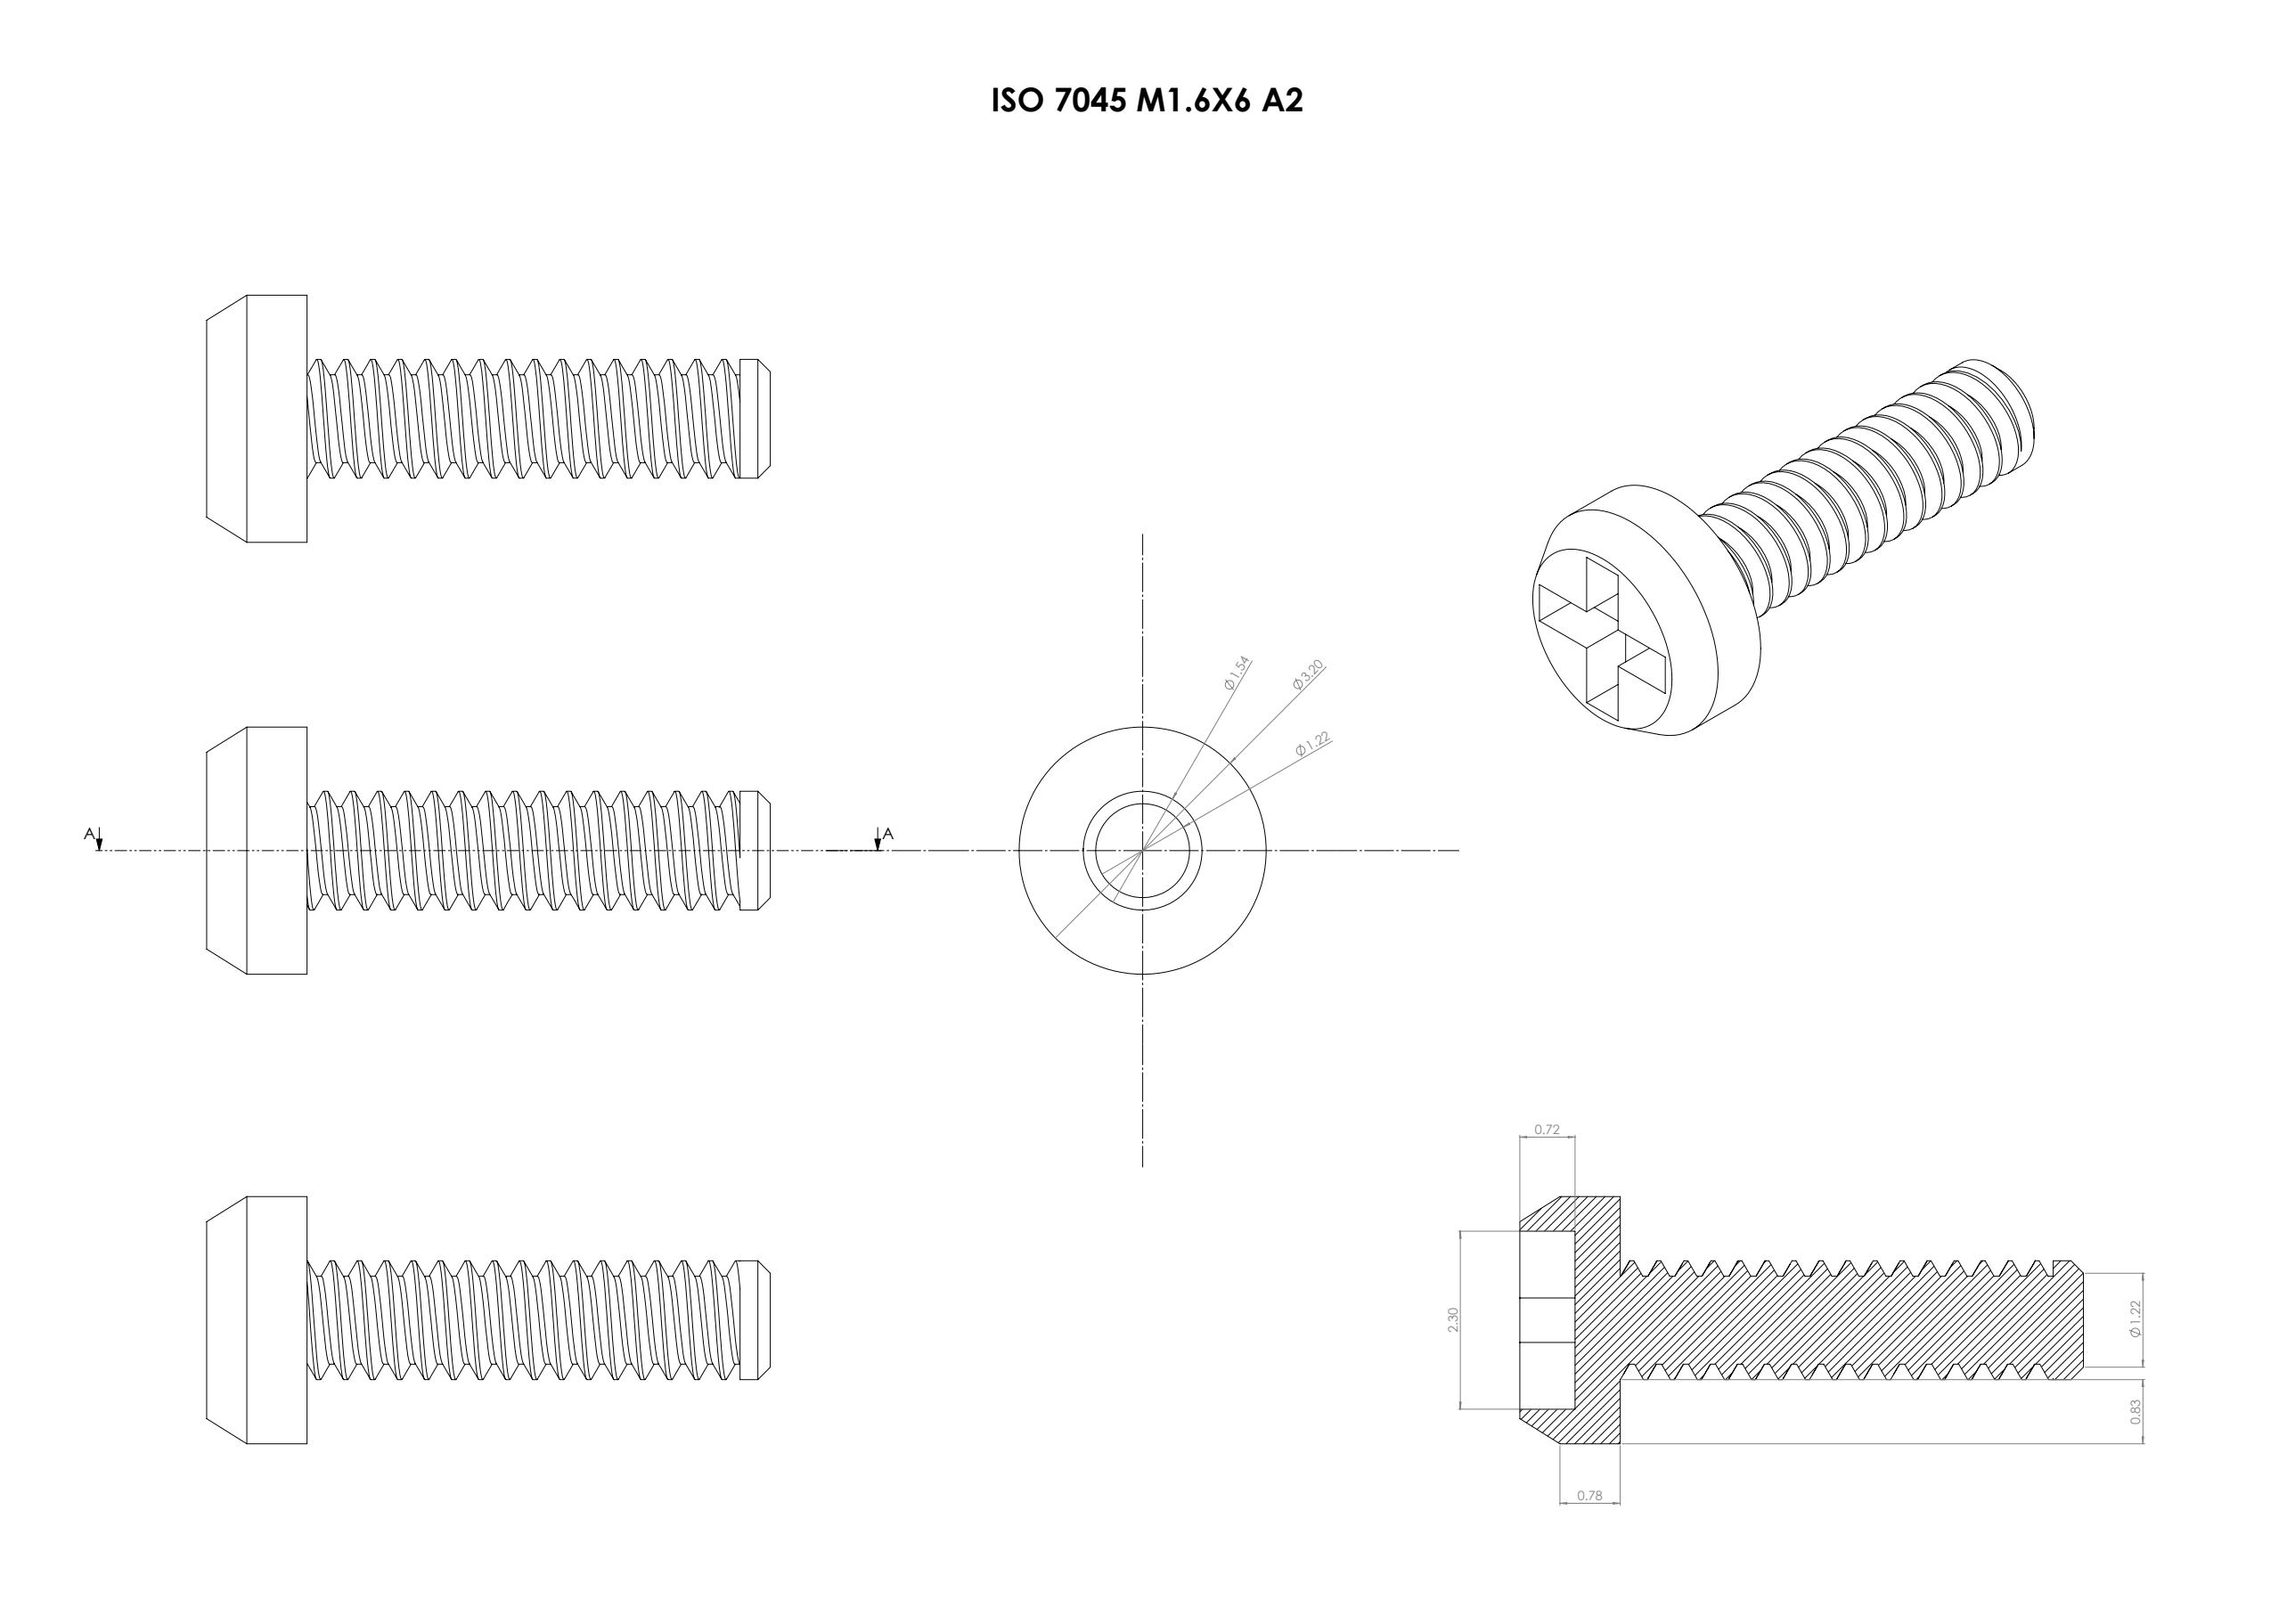
ISO-10303-21;
HEADER;
/* Generated by software containing ST-Developer
 * from STEP Tools, Inc. (www.steptools.com) 
 */

FILE_DESCRIPTION(
/* description */ (''),
/* implementation_level */ '2;1');

FILE_NAME(
/* name */ '19_ISO_7045_M1.6x6_A2.step',
/* time_stamp */ '2026-10-19T23:00:43-07:00',
/* author */ (''),
/* organization */ (''),
/* preprocessor_version */ 'ST-DEVELOPER v20.2',
/* originating_system */ 'Autodesk Translation Framework v15.15.0.0',
/* authorisation */ '');

FILE_SCHEMA (('AUTOMOTIVE_DESIGN { 1 0 10303 214 3 1 1 }'));
ENDSEC;

DATA;
#10=MECHANICAL_DESIGN_GEOMETRIC_PRESENTATION_REPRESENTATION('',(#1015),#55002);
#482=B_SPLINE_SURFACE_WITH_KNOTS('',3,3,((#53741,#53742,#53743,#53744,#53745,
#53746,#53747,#53748,#53749,#53750,#53751,#53752,#53753,#53754,#53755,#53756,
#53757,#53758,#53759,#53760,#53761,#53762,#53763,#53764,#53765,#53766,#53767,
#53768,#53769,#53770,#53771,#53772,#53773,#53774,#53775,#53776,#53777,#53778,
#53779,#53780,#53781,#53782,#53783,#53784,#53785,#53786,#53787,#53788,#53789,
#53790,#53791,#53792,#53793,#53794,#53795,#53796,#53797,#53798,#53799,#53800,
#53801,#53802,#53803,#53804,#53805,#53806,#53807,#53808,#53809,#53810,#53811,
#53812,#53813,#53814,#53815,#53816,#53817,#53818,#53819,#53820,#53821,#53822,
#53823,#53824,#53825,#53826,#53827,#53828,#53829,#53830,#53831,#53832,#53833,
#53834,#53835,#53836,#53837,#53838,#53839,#53840,#53841,#53842,#53843,#53844,
#53845,#53846),(#53847,#53848,#53849,#53850,#53851,#53852,#53853,#53854,
#53855,#53856,#53857,#53858,#53859,#53860,#53861,#53862,#53863,#53864,#53865,
#53866,#53867,#53868,#53869,#53870,#53871,#53872,#53873,#53874,#53875,#53876,
#53877,#53878,#53879,#53880,#53881,#53882,#53883,#53884,#53885,#53886,#53887,
#53888,#53889,#53890,#53891,#53892,#53893,#53894,#53895,#53896,#53897,#53898,
#53899,#53900,#53901,#53902,#53903,#53904,#53905,#53906,#53907,#53908,#53909,
#53910,#53911,#53912,#53913,#53914,#53915,#53916,#53917,#53918,#53919,#53920,
#53921,#53922,#53923,#53924,#53925,#53926,#53927,#53928,#53929,#53930,#53931,
#53932,#53933,#53934,#53935,#53936,#53937,#53938,#53939,#53940,#53941,#53942,
#53943,#53944,#53945,#53946,#53947,#53948,#53949,#53950,#53951,#53952),
(#53953,#53954,#53955,#53956,#53957,#53958,#53959,#53960,#53961,#53962,
#53963,#53964,#53965,#53966,#53967,#53968,#53969,#53970,#53971,#53972,#53973,
#53974,#53975,#53976,#53977,#53978,#53979,#53980,#53981,#53982,#53983,#53984,
#53985,#53986,#53987,#53988,#53989,#53990,#53991,#53992,#53993,#53994,#53995,
#53996,#53997,#53998,#53999,#54000,#54001,#54002,#54003,#54004,#54005,#54006,
#54007,#54008,#54009,#54010,#54011,#54012,#54013,#54014,#54015,#54016,#54017,
#54018,#54019,#54020,#54021,#54022,#54023,#54024,#54025,#54026,#54027,#54028,
#54029,#54030,#54031,#54032,#54033,#54034,#54035,#54036,#54037,#54038,#54039,
#54040,#54041,#54042,#54043,#54044,#54045,#54046,#54047,#54048,#54049,#54050,
#54051,#54052,#54053,#54054,#54055,#54056,#54057,#54058),(#54059,#54060,
#54061,#54062,#54063,#54064,#54065,#54066,#54067,#54068,#54069,#54070,#54071,
#54072,#54073,#54074,#54075,#54076,#54077,#54078,#54079,#54080,#54081,#54082,
#54083,#54084,#54085,#54086,#54087,#54088,#54089,#54090,#54091,#54092,#54093,
#54094,#54095,#54096,#54097,#54098,#54099,#54100,#54101,#54102,#54103,#54104,
#54105,#54106,#54107,#54108,#54109,#54110,#54111,#54112,#54113,#54114,#54115,
#54116,#54117,#54118,#54119,#54120,#54121,#54122,#54123,#54124,#54125,#54126,
#54127,#54128,#54129,#54130,#54131,#54132,#54133,#54134,#54135,#54136,#54137,
#54138,#54139,#54140,#54141,#54142,#54143,#54144,#54145,#54146,#54147,#54148,
#54149,#54150,#54151,#54152,#54153,#54154,#54155,#54156,#54157,#54158,#54159,
#54160,#54161,#54162,#54163,#54164)),.UNSPECIFIED.,.F.,.F.,.F.,(4,4),(4,
1,1,1,1,1,1,1,1,1,1,1,1,1,1,1,1,1,1,1,1,1,1,1,1,1,1,1,1,1,1,1,1,1,1,1,1,
1,1,1,1,1,1,1,1,1,1,1,1,1,1,1,1,1,1,1,1,1,1,1,1,1,1,1,1,1,1,1,1,1,1,1,1,
1,1,1,1,1,1,1,1,1,1,1,1,1,1,1,1,1,1,1,1,1,1,1,1,1,1,1,1,1,1,4),(0.,0.0230940107675851),
(12.4478189520753,13.4453674388536,14.4429159256318,15.4404644124101,16.4380128991884,
17.4355613859667,18.433109872745,19.4306583595232,20.4282068463015,21.4257553330798,
22.423303819858,23.4208523066363,24.4184007934146,25.4159492801929,26.4134977669712,
27.4110462537494,28.4085947405277,29.406143227306,30.4036917140842,31.4012402008625,
32.3987886876408,33.3963371744191,34.3938856611974,35.3914341479756,36.3889826347539,
37.3865311215322,38.3840796083105,39.3816280950887,40.379176581867,41.3767250686453,
42.3742735554236,43.3718220422018,44.3693705289801,45.3669190157584,46.3644675025367,
47.3620159893149,48.3595644760932,49.3571129628715,50.3546614496498,51.352209936428,
52.3497584232063,53.3473069099846,54.3448553967629,55.3424038835411,56.3399523703194,
57.3375008570977,58.335049343876,59.3325978306542,60.3301463174325,61.3276948042108,
62.3252432909891,63.3227917777673,64.3203402645456,65.3178887513239,66.3154372381021,
67.3129857248804,68.3105342116587,69.308082698437,70.3056311852153,71.3031796719935,
72.3007281587718,73.2982766455501,74.2958251323284,75.2933736191066,76.2909221058849,
77.2884705926632,78.2860190794415,79.2835675662197,80.281116052998,81.2786645397763,
82.2762130265546,83.2737615133328,84.2713100001111,85.2688584868894,86.2664069736677,
87.2639554604459,88.2615039472242,89.2590524340025,90.2566009207808,91.254149407559,
92.2516978943373,93.2492463811156,94.2467948678939,95.2443433546721,96.2418918414504,
97.2394403282287,98.236988815007,99.2345373017852,100.232085788564,101.229634275342,
102.22718276212,103.224731248898,104.222279735677,105.219828222455,106.217376709233,
107.214925196011,108.21247368279,109.210022169568,110.207570656346,111.205119143125,
112.202667629903,113.200216116681,114.197764603459,115.195313090238),
 .UNSPECIFIED.);
#483=B_SPLINE_SURFACE_WITH_KNOTS('',3,3,((#54329,#54330,#54331,#54332,#54333,
#54334,#54335,#54336,#54337,#54338,#54339,#54340,#54341,#54342,#54343,#54344,
#54345,#54346,#54347,#54348,#54349,#54350,#54351,#54352,#54353,#54354,#54355,
#54356,#54357,#54358,#54359,#54360,#54361,#54362,#54363,#54364,#54365,#54366,
#54367,#54368,#54369,#54370,#54371,#54372,#54373,#54374,#54375,#54376,#54377,
#54378,#54379,#54380,#54381,#54382,#54383,#54384,#54385,#54386,#54387,#54388,
#54389,#54390,#54391,#54392,#54393,#54394,#54395,#54396,#54397,#54398,#54399,
#54400,#54401,#54402,#54403,#54404,#54405,#54406,#54407,#54408,#54409,#54410,
#54411,#54412,#54413,#54414,#54415,#54416,#54417,#54418,#54419,#54420,#54421,
#54422,#54423,#54424,#54425,#54426,#54427,#54428,#54429,#54430,#54431,#54432,
#54433,#54434),(#54435,#54436,#54437,#54438,#54439,#54440,#54441,#54442,
#54443,#54444,#54445,#54446,#54447,#54448,#54449,#54450,#54451,#54452,#54453,
#54454,#54455,#54456,#54457,#54458,#54459,#54460,#54461,#54462,#54463,#54464,
#54465,#54466,#54467,#54468,#54469,#54470,#54471,#54472,#54473,#54474,#54475,
#54476,#54477,#54478,#54479,#54480,#54481,#54482,#54483,#54484,#54485,#54486,
#54487,#54488,#54489,#54490,#54491,#54492,#54493,#54494,#54495,#54496,#54497,
#54498,#54499,#54500,#54501,#54502,#54503,#54504,#54505,#54506,#54507,#54508,
#54509,#54510,#54511,#54512,#54513,#54514,#54515,#54516,#54517,#54518,#54519,
#54520,#54521,#54522,#54523,#54524,#54525,#54526,#54527,#54528,#54529,#54530,
#54531,#54532,#54533,#54534,#54535,#54536,#54537,#54538,#54539,#54540),
(#54541,#54542,#54543,#54544,#54545,#54546,#54547,#54548,#54549,#54550,
#54551,#54552,#54553,#54554,#54555,#54556,#54557,#54558,#54559,#54560,#54561,
#54562,#54563,#54564,#54565,#54566,#54567,#54568,#54569,#54570,#54571,#54572,
#54573,#54574,#54575,#54576,#54577,#54578,#54579,#54580,#54581,#54582,#54583,
#54584,#54585,#54586,#54587,#54588,#54589,#54590,#54591,#54592,#54593,#54594,
#54595,#54596,#54597,#54598,#54599,#54600,#54601,#54602,#54603,#54604,#54605,
#54606,#54607,#54608,#54609,#54610,#54611,#54612,#54613,#54614,#54615,#54616,
#54617,#54618,#54619,#54620,#54621,#54622,#54623,#54624,#54625,#54626,#54627,
#54628,#54629,#54630,#54631,#54632,#54633,#54634,#54635,#54636,#54637,#54638,
#54639,#54640,#54641,#54642,#54643,#54644,#54645,#54646),(#54647,#54648,
#54649,#54650,#54651,#54652,#54653,#54654,#54655,#54656,#54657,#54658,#54659,
#54660,#54661,#54662,#54663,#54664,#54665,#54666,#54667,#54668,#54669,#54670,
#54671,#54672,#54673,#54674,#54675,#54676,#54677,#54678,#54679,#54680,#54681,
#54682,#54683,#54684,#54685,#54686,#54687,#54688,#54689,#54690,#54691,#54692,
#54693,#54694,#54695,#54696,#54697,#54698,#54699,#54700,#54701,#54702,#54703,
#54704,#54705,#54706,#54707,#54708,#54709,#54710,#54711,#54712,#54713,#54714,
#54715,#54716,#54717,#54718,#54719,#54720,#54721,#54722,#54723,#54724,#54725,
#54726,#54727,#54728,#54729,#54730,#54731,#54732,#54733,#54734,#54735,#54736,
#54737,#54738,#54739,#54740,#54741,#54742,#54743,#54744,#54745,#54746,#54747,
#54748,#54749,#54750,#54751,#54752)),.UNSPECIFIED.,.F.,.F.,.F.,(4,4),(4,
1,1,1,1,1,1,1,1,1,1,1,1,1,1,1,1,1,1,1,1,1,1,1,1,1,1,1,1,1,1,1,1,1,1,1,1,
1,1,1,1,1,1,1,1,1,1,1,1,1,1,1,1,1,1,1,1,1,1,1,1,1,1,1,1,1,1,1,1,1,1,1,1,
1,1,1,1,1,1,1,1,1,1,1,1,1,1,1,1,1,1,1,1,1,1,1,1,1,1,1,1,1,1,4),(0.,0.0230940107675851),
(15.755244690395,16.7527931771733,17.7503416639516,18.7478901507299,19.7454386375081,
20.7429871242864,21.7405356110647,22.738084097843,23.7356325846212,24.7331810713995,
25.7307295581778,26.7282780449561,27.7258265317343,28.7233750185126,29.7209235052909,
30.7184719920692,31.7160204788475,32.7135689656257,33.711117452404,34.7086659391823,
35.7062144259606,36.7037629127388,37.7013113995171,38.6988598862954,39.6964083730737,
40.6939568598519,41.6915053466302,42.6890538334085,43.6866023201868,44.684150806965,
45.6816992937433,46.6792477805216,47.6767962672999,48.6743447540781,49.6718932408564,
50.6694417276347,51.666990214413,52.6645387011912,53.6620871879695,54.6596356747478,
55.6571841615261,56.6547326483043,57.6522811350826,58.6498296218609,59.6473781086392,
60.6449265954174,61.6424750821957,62.640023568974,63.6375720557523,64.6351205425305,
65.6326690293088,66.6302175160871,67.6277660028654,68.6253144896436,69.6228629764219,
70.6204114632002,71.6179599499785,72.6155084367567,73.613056923535,74.6106054103133,
75.6081538970916,76.6057023838698,77.6032508706481,78.6007993574264,79.5983478442047,
80.595896330983,81.5934448177612,82.5909933045395,83.5885417913178,84.5860902780961,
85.5836387648743,86.5811872516526,87.5787357384309,88.5762842252092,89.5738327119874,
90.5713811987657,91.568929685544,92.5664781723222,93.5640266591005,94.5615751458788,
95.5591236326571,96.5566721194354,97.5542206062136,98.5517690929919,99.5493175797702,
100.546866066548,101.544414553327,102.541963040105,103.539511526883,104.537060013662,
105.53460850044,106.532156987218,107.529705473996,108.527253960775,109.524802447553,
110.522350934331,111.519899421109,112.517447907888,113.514996394666,114.512544881444,
115.510093368223,116.507641855001,117.505190341779,118.502738828557),
 .UNSPECIFIED.);
#882=B_SPLINE_CURVE_WITH_KNOTS('',3,(#52556,#52557,#52558,#52559,#52560,
#52561,#52562,#52563,#52564,#52565,#52566,#52567,#52568,#52569,#52570,#52571),
 .UNSPECIFIED.,.F.,.F.,(4,3,3,3,3,4),(-6.23590388473343,-5.98529092066965,
-4.98774243389138,-3.9901939471131,-2.99264546033482,-2.07291355912486),
 .UNSPECIFIED.);
#883=B_SPLINE_CURVE_WITH_KNOTS('',3,(#52579,#52580,#52581,#52582,#52583,
#52584,#52585,#52586,#52587,#52588,#52589,#52590,#52591),.UNSPECIFIED.,
 .F.,.F.,(4,3,3,3,4),(0.,0.997548486778257,1.99509697355654,2.99264546033483,
3.26014431587347),.UNSPECIFIED.);
#884=B_SPLINE_CURVE_WITH_KNOTS('',3,(#52596,#52597,#52598,#52599,#52600,
#52601,#52602,#52603,#52604,#52605,#52606,#52607,#52608,#52609,#52610,#52611,
#52612,#52613,#52614,#52615,#52616,#52617),.UNSPECIFIED.,.F.,.F.,(4,3,3,
3,3,3,3,4),(-12.519089191913,-11.9705818413393,-10.973033354561,-9.97548486778276,
-8.97793638100448,-7.9803878942262,-6.98283940744793,-6.23590388473343),
 .UNSPECIFIED.);
#885=B_SPLINE_CURVE_WITH_KNOTS('',3,(#52618,#52619,#52620,#52621,#52622,
#52623,#52624,#52625,#52626,#52627,#52628,#52629,#52630,#52631,#52632,#52633,
#52634,#52635,#52636,#52637,#52638,#52639),.UNSPECIFIED.,.F.,.F.,(4,3,3,
3,3,3,3,4),(3.26014431587347,3.99019394711311,4.98774243389138,5.98529092066965,
6.98283940744792,7.9803878942262,8.97793638100447,9.54332962305307),
 .UNSPECIFIED.);
#886=B_SPLINE_CURVE_WITH_KNOTS('',3,(#52644,#52645,#52646,#52647,#52648,
#52649,#52650,#52651,#52652,#52653,#52654,#52655,#52656,#52657,#52658,#52659,
#52660,#52661,#52662,#52663,#52664,#52665),.UNSPECIFIED.,.F.,.F.,(4,3,3,
3,3,3,3,4),(-18.8022744990926,-17.955872762009,-16.9583242752307,-15.9607757884524,
-14.9632273016741,-13.9656788148959,-12.9681303281176,-12.519089191913),
 .UNSPECIFIED.);
#887=B_SPLINE_CURVE_WITH_KNOTS('',3,(#52666,#52667,#52668,#52669,#52670,
#52671,#52672,#52673,#52674,#52675,#52676,#52677,#52678,#52679,#52680,#52681,
#52682,#52683,#52684,#52685,#52686,#52687),.UNSPECIFIED.,.F.,.F.,(4,3,3,
3,3,3,3,4),(9.54332962305307,9.97548486778275,10.973033354561,11.9705818413393,
12.9681303281176,13.9656788148959,14.9632273016741,15.8265149302327),
 .UNSPECIFIED.);
#888=B_SPLINE_CURVE_WITH_KNOTS('',3,(#52692,#52693,#52694,#52695,#52696,
#52697,#52698,#52699,#52700,#52701,#52702,#52703,#52704,#52705,#52706,#52707,
#52708,#52709,#52710,#52711,#52712,#52713,#52714,#52715,#52716),
 .UNSPECIFIED.,.F.,.F.,(4,3,3,3,3,3,3,3,4),(-25.0854598062722,-24.9387121694569,
-23.9411636826786,-22.9436151959003,-21.9460667091221,-20.9485182223438,
-19.9509697355655,-18.9534212487872,-18.8022744990926),.UNSPECIFIED.);
#889=B_SPLINE_CURVE_WITH_KNOTS('',3,(#52717,#52718,#52719,#52720,#52721,
#52722,#52723,#52724,#52725,#52726,#52727,#52728,#52729,#52730,#52731,#52732,
#52733,#52734,#52735,#52736,#52737,#52738,#52739,#52740,#52741),
 .UNSPECIFIED.,.F.,.F.,(4,3,3,3,3,3,3,3,4),(15.8265149302327,15.9607757884524,
16.9583242752307,17.955872762009,18.9534212487872,19.9509697355655,20.9485182223438,
21.9460667091221,22.1097002374122),.UNSPECIFIED.);
#890=B_SPLINE_CURVE_WITH_KNOTS('',3,(#52746,#52747,#52748,#52749,#52750,
#52751,#52752,#52753,#52754,#52755,#52756,#52757,#52758,#52759,#52760,#52761,
#52762,#52763,#52764,#52765,#52766,#52767),.UNSPECIFIED.,.F.,.F.,(4,3,3,
3,3,3,3,4),(-31.3686451134518,-30.9240030901265,-29.9264546033483,-28.92890611657,
-27.9313576297917,-26.9338091430134,-25.9362606562352,-25.0854598062722),
 .UNSPECIFIED.);
#891=B_SPLINE_CURVE_WITH_KNOTS('',3,(#52768,#52769,#52770,#52771,#52772,
#52773,#52774,#52775,#52776,#52777,#52778,#52779,#52780,#52781,#52782,#52783,
#52784,#52785,#52786,#52787,#52788,#52789),.UNSPECIFIED.,.F.,.F.,(4,3,3,
3,3,3,3,4),(22.1097002374122,22.9436151959003,23.9411636826786,24.9387121694569,
25.9362606562352,26.9338091430134,27.9313576297917,28.3928855445918),
 .UNSPECIFIED.);
#892=B_SPLINE_CURVE_WITH_KNOTS('',3,(#52794,#52795,#52796,#52797,#52798,
#52799,#52800,#52801,#52802,#52803,#52804,#52805,#52806,#52807,#52808,#52809,
#52810,#52811,#52812,#52813,#52814,#52815),.UNSPECIFIED.,.F.,.F.,(4,3,3,
3,3,3,3,4),(-37.6518304206314,-36.9092940107962,-35.9117455240179,-34.9141970372396,
-33.9166485504614,-32.9191000636831,-31.9215515769048,-31.3686451134518),
 .UNSPECIFIED.);
#893=B_SPLINE_CURVE_WITH_KNOTS('',3,(#52816,#52817,#52818,#52819,#52820,
#52821,#52822,#52823,#52824,#52825,#52826,#52827,#52828,#52829,#52830,#52831,
#52832,#52833,#52834,#52835,#52836,#52837),.UNSPECIFIED.,.F.,.F.,(4,3,3,
3,3,3,3,4),(28.3928855445918,28.92890611657,29.9264546033483,30.9240030901265,
31.9215515769048,32.9191000636831,33.9166485504614,34.6760708517714),
 .UNSPECIFIED.);
#894=B_SPLINE_CURVE_WITH_KNOTS('',3,(#52842,#52843,#52844,#52845,#52846,
#52847,#52848,#52849,#52850,#52851,#52852,#52853,#52854,#52855,#52856,#52857,
#52858,#52859,#52860,#52861,#52862,#52863,#52864,#52865,#52866),
 .UNSPECIFIED.,.F.,.F.,(4,3,3,3,3,3,3,3,4),(-43.9350157278109,-43.8921334182441,
-42.8945849314659,-41.8970364446876,-40.8994879579093,-39.901939471131,
-38.9043909843527,-37.9068424975745,-37.6518304206314),.UNSPECIFIED.);
#895=B_SPLINE_CURVE_WITH_KNOTS('',3,(#52867,#52868,#52869,#52870,#52871,
#52872,#52873,#52874,#52875,#52876,#52877,#52878,#52879,#52880,#52881,#52882,
#52883,#52884,#52885,#52886,#52887,#52888,#52889,#52890,#52891),
 .UNSPECIFIED.,.F.,.F.,(4,3,3,3,3,3,3,3,4),(34.6760708517714,34.9141970372396,
35.9117455240179,36.9092940107962,37.9068424975745,38.9043909843527,39.901939471131,
40.8994879579093,40.959256158951),.UNSPECIFIED.);
#896=B_SPLINE_CURVE_WITH_KNOTS('',3,(#52896,#52897,#52898,#52899,#52900,
#52901,#52902,#52903,#52904,#52905,#52906,#52907,#52908,#52909,#52910,#52911,
#52912,#52913,#52914,#52915,#52916,#52917),.UNSPECIFIED.,.F.,.F.,(4,3,3,
3,3,3,3,4),(-50.2182010349905,-49.8774243389138,-48.8798758521355,-47.8823273653572,
-46.8847788785789,-45.8872303918007,-44.8896819050224,-43.9350157278109),
 .UNSPECIFIED.);
#897=B_SPLINE_CURVE_WITH_KNOTS('',3,(#52918,#52919,#52920,#52921,#52922,
#52923,#52924,#52925,#52926,#52927,#52928,#52929,#52930,#52931,#52932,#52933,
#52934,#52935,#52936,#52937,#52938,#52939),.UNSPECIFIED.,.F.,.F.,(4,3,3,
3,3,3,3,4),(40.959256158951,41.8970364446876,42.8945849314658,43.8921334182441,
44.8896819050224,45.8872303918007,46.8847788785789,47.2424414661306),
 .UNSPECIFIED.);
#898=B_SPLINE_CURVE_WITH_KNOTS('',3,(#52944,#52945,#52946,#52947,#52948,
#52949,#52950,#52951,#52952,#52953,#52954,#52955,#52956,#52957,#52958,#52959,
#52960,#52961,#52962,#52963,#52964,#52965),.UNSPECIFIED.,.F.,.F.,(4,3,3,
3,3,3,3,4),(-56.5013863421701,-55.8627152595834,-54.8651667728052,-53.8676182860269,
-52.8700697992486,-51.8725213124703,-50.874972825692,-50.2182010349905),
 .UNSPECIFIED.);
#899=B_SPLINE_CURVE_WITH_KNOTS('',3,(#52966,#52967,#52968,#52969,#52970,
#52971,#52972,#52973,#52974,#52975,#52976,#52977,#52978,#52979,#52980,#52981,
#52982,#52983,#52984,#52985,#52986,#52987),.UNSPECIFIED.,.F.,.F.,(4,3,3,
3,3,3,3,4),(47.2424414661306,47.8823273653572,48.8798758521355,49.8774243389137,
50.874972825692,51.8725213124703,52.8700697992486,53.5256267733102),
 .UNSPECIFIED.);
#900=B_SPLINE_CURVE_WITH_KNOTS('',3,(#52992,#52993,#52994,#52995,#52996,
#52997,#52998,#52999,#53000,#53001,#53002,#53003,#53004,#53005,#53006,#53007,
#53008,#53009,#53010,#53011,#53012,#53013),.UNSPECIFIED.,.F.,.F.,(4,3,3,
3,3,3,3,4),(-62.7845716493497,-61.8480061802531,-60.8504576934748,-59.8529092066965,
-58.8553607199183,-57.85781223314,-56.8602637463617,-56.5013863421701),
 .UNSPECIFIED.);
#901=B_SPLINE_CURVE_WITH_KNOTS('',3,(#53014,#53015,#53016,#53017,#53018,
#53019,#53020,#53021,#53022,#53023,#53024,#53025,#53026,#53027,#53028,#53029,
#53030,#53031,#53032,#53033,#53034,#53035),.UNSPECIFIED.,.F.,.F.,(4,3,3,
3,3,3,3,4),(53.5256267733102,53.8676182860269,54.8651667728051,55.8627152595834,
56.8602637463617,57.85781223314,58.8553607199182,59.8088120804898),
 .UNSPECIFIED.);
#902=B_SPLINE_CURVE_WITH_KNOTS('',3,(#53040,#53041,#53042,#53043,#53044,
#53045,#53046,#53047,#53048,#53049,#53050,#53051,#53052,#53053,#53054,#53055,
#53056,#53057,#53058,#53059,#53060,#53061,#53062,#53063,#53064),
 .UNSPECIFIED.,.F.,.F.,(4,3,3,3,3,3,3,3,4),(-69.0677569565293,-68.830845587701,
-67.8332971009227,-66.8357486141444,-65.8382001273662,-64.8406516405879,
-63.8431031538096,-62.8455546670314,-62.7845716493497),.UNSPECIFIED.);
#903=B_SPLINE_CURVE_WITH_KNOTS('',3,(#53065,#53066,#53067,#53068,#53069,
#53070,#53071,#53072,#53073,#53074,#53075,#53076,#53077,#53078,#53079,#53080,
#53081,#53082,#53083,#53084,#53085,#53086,#53087,#53088,#53089),
 .UNSPECIFIED.,.F.,.F.,(4,3,3,3,3,3,3,3,4),(59.8088120804898,59.8529092066965,
60.8504576934748,61.8480061802531,62.8455546670313,63.8431031538096,64.8406516405879,
65.8382001273662,66.0919973876694),.UNSPECIFIED.);
#904=B_SPLINE_CURVE_WITH_KNOTS('',3,(#53094,#53095,#53096,#53097,#53098,
#53099,#53100,#53101,#53102,#53103,#53104,#53105,#53106,#53107,#53108,#53109,
#53110,#53111,#53112,#53113,#53114,#53115),.UNSPECIFIED.,.F.,.F.,(4,3,3,
3,3,3,3,4),(-75.3509422637089,-74.8161365083707,-73.8185880215924,-72.8210395348141,
-71.8234910480358,-70.8259425612576,-69.8283940744793,-69.0677569565293),
 .UNSPECIFIED.);
#905=B_SPLINE_CURVE_WITH_KNOTS('',3,(#53116,#53117,#53118,#53119,#53120,
#53121,#53122,#53123,#53124,#53125,#53126,#53127,#53128,#53129,#53130,#53131,
#53132,#53133,#53134,#53135,#53136,#53137),.UNSPECIFIED.,.F.,.F.,(4,3,3,
3,3,3,3,4),(66.0919973876694,66.8357486141444,67.8332971009227,68.830845587701,
69.8283940744792,70.8259425612575,71.8234910480358,72.375182694849),
 .UNSPECIFIED.);
#906=B_SPLINE_CURVE_WITH_KNOTS('',3,(#53142,#53143,#53144,#53145,#53146,
#53147,#53148,#53149,#53150,#53151,#53152,#53153,#53154,#53155,#53156,#53157,
#53158,#53159,#53160,#53161,#53162,#53163),.UNSPECIFIED.,.F.,.F.,(4,3,3,
3,3,3,3,4),(-81.6341275708885,-80.8014274290403,-79.803878942262,-78.8063304554838,
-77.8087819687055,-76.8112334819272,-75.8136849951489,-75.3509422637089),
 .UNSPECIFIED.);
#907=B_SPLINE_CURVE_WITH_KNOTS('',3,(#53164,#53165,#53166,#53167,#53168,
#53169,#53170,#53171,#53172,#53173,#53174,#53175,#53176,#53177,#53178,#53179,
#53180,#53181,#53182,#53183,#53184,#53185),.UNSPECIFIED.,.F.,.F.,(4,3,3,
3,3,3,3,4),(72.375182694849,72.8210395348141,73.8185880215924,74.8161365083706,
75.8136849951489,76.8112334819272,77.8087819687055,78.6583680020286),
 .UNSPECIFIED.);
#908=B_SPLINE_CURVE_WITH_KNOTS('',3,(#53190,#53191,#53192,#53193,#53194,
#53195,#53196,#53197,#53198,#53199,#53200,#53201,#53202,#53203,#53204,#53205,
#53206,#53207,#53208,#53209,#53210,#53211,#53212,#53213,#53214),
 .UNSPECIFIED.,.F.,.F.,(4,3,3,3,3,3,3,3,4),(-87.9173128780681,-87.7842668364882,
-86.78671834971,-85.7891698629317,-84.7916213761534,-83.7940728893752,-82.7965244025969,
-81.7989759158186,-81.6341275708885),.UNSPECIFIED.);
#909=B_SPLINE_CURVE_WITH_KNOTS('',3,(#53215,#53216,#53217,#53218,#53219,
#53220,#53221,#53222,#53223,#53224,#53225,#53226,#53227,#53228,#53229,#53230,
#53231,#53232,#53233,#53234,#53235,#53236,#53237,#53238,#53239),
 .UNSPECIFIED.,.F.,.F.,(4,3,3,3,3,3,3,3,4),(78.6583680020286,78.8063304554837,
79.803878942262,80.8014274290403,81.7989759158185,82.7965244025968,83.7940728893751,
84.7916213761534,84.9415533092082),.UNSPECIFIED.);
#910=B_SPLINE_CURVE_WITH_KNOTS('',3,(#53244,#53245,#53246,#53247,#53248,
#53249,#53250,#53251,#53252,#53253,#53254,#53255,#53256,#53257,#53258,#53259,
#53260,#53261,#53262,#53263,#53264,#53265),.UNSPECIFIED.,.F.,.F.,(4,3,3,
3,3,3,3,4),(-94.2004981852477,-93.7695577571579,-92.7720092703796,-91.7744607836013,
-90.7769122968231,-89.7793638100448,-88.7818153232665,-87.9173128780681),
 .UNSPECIFIED.);
#911=B_SPLINE_CURVE_WITH_KNOTS('',3,(#53266,#53267,#53268,#53269,#53270,
#53271,#53272,#53273,#53274,#53275,#53276,#53277,#53278,#53279,#53280,#53281,
#53282,#53283,#53284,#53285,#53286,#53287),.UNSPECIFIED.,.F.,.F.,(4,3,3,
3,3,3,3,4),(84.9415533092082,85.7891698629316,86.7867183497099,87.7842668364882,
88.7818153232665,89.7793638100448,90.776912296823,91.2247386163878),
 .UNSPECIFIED.);
#912=B_SPLINE_CURVE_WITH_KNOTS('',3,(#53292,#53293,#53294,#53295,#53296,
#53297,#53298,#53299,#53300,#53301,#53302,#53303,#53304,#53305,#53306,#53307,
#53308,#53309,#53310,#53311,#53312,#53313),.UNSPECIFIED.,.F.,.F.,(4,3,3,
3,3,3,3,4),(-100.483683492427,-99.7548486778276,-98.7573001910493,-97.759751704271,
-96.7622032174927,-95.7646547307145,-94.7671062439362,-94.2004981852477),
 .UNSPECIFIED.);
#913=B_SPLINE_CURVE_WITH_KNOTS('',3,(#53314,#53315,#53316,#53317,#53318,
#53319,#53320,#53321,#53322,#53323,#53324,#53325,#53326,#53327,#53328,#53329,
#53330,#53331,#53332,#53333,#53334,#53335),.UNSPECIFIED.,.F.,.F.,(4,3,3,
3,3,3,3,4),(91.2247386163878,91.7744607836013,92.7720092703796,93.7695577571579,
94.7671062439361,95.7646547307144,96.7622032174927,97.5079239235673),
 .UNSPECIFIED.);
#914=B_SPLINE_CURVE_WITH_KNOTS('',3,(#53341,#53342,#53343,#53344),
 .UNSPECIFIED.,.F.,.F.,(4,4),(116.238928182822,116.429825269433),
 .UNSPECIFIED.);
#915=B_SPLINE_CURVE_WITH_KNOTS('',3,(#53350,#53351,#53352,#53353,#53354,
#53355,#53356,#53357,#53358,#53359),.UNSPECIFIED.,.F.,.F.,(4,1,1,1,1,1,
1,4),(109.955742875643,110.522350934331,111.519899421109,112.517447907888,
113.514996394666,114.512544881444,115.510093368223,116.238928182822),
 .UNSPECIFIED.);
#916=B_SPLINE_CURVE_WITH_KNOTS('',3,(#53362,#53363,#53364,#53365,#53366,
#53367,#53368,#53369,#53370),.UNSPECIFIED.,.F.,.F.,(4,1,1,1,1,1,4),(109.955742875643,
110.207570656346,111.205119143125,112.202667629903,113.200216116681,114.197764603459,
115.195313090238),.UNSPECIFIED.);
#917=B_SPLINE_CURVE_WITH_KNOTS('',3,(#53375,#53376,#53377,#53378,#53379,
#53380,#53381,#53382,#53383,#53384),.UNSPECIFIED.,.F.,.F.,(4,1,1,1,1,1,
1,4),(103.672557568463,104.537060013662,105.53460850044,106.532156987218,
107.529705473996,108.527253960775,109.524802447553,109.955742875643),
 .UNSPECIFIED.);
#918=B_SPLINE_CURVE_WITH_KNOTS('',3,(#53385,#53386,#53387,#53388,#53389,
#53390,#53391,#53392,#53393,#53394),.UNSPECIFIED.,.F.,.F.,(4,1,1,1,1,1,
1,4),(103.672557568463,104.222279735677,105.219828222455,106.217376709233,
107.214925196011,108.21247368279,109.210022169568,109.955742875643),
 .UNSPECIFIED.);
#919=B_SPLINE_CURVE_WITH_KNOTS('',3,(#53399,#53400,#53401,#53402,#53403,
#53404,#53405,#53406,#53407,#53408,#53409),.UNSPECIFIED.,.F.,.F.,(4,1,1,
1,1,1,1,1,4),(97.3893722612836,97.5542206062136,98.5517690929919,99.5493175797702,
100.546866066548,101.544414553327,102.541963040105,103.539511526883,103.672557568463),
 .UNSPECIFIED.);
#920=B_SPLINE_CURVE_WITH_KNOTS('',3,(#53410,#53411,#53412,#53413,#53414,
#53415,#53416,#53417,#53418,#53419),.UNSPECIFIED.,.F.,.F.,(4,1,1,1,1,1,
1,4),(97.3893722612836,98.236988815007,99.2345373017852,100.232085788564,
101.229634275342,102.22718276212,103.224731248898,103.672557568463),
 .UNSPECIFIED.);
#921=B_SPLINE_CURVE_WITH_KNOTS('',3,(#53424,#53425,#53426,#53427,#53428,
#53429,#53430,#53431,#53432,#53433),.UNSPECIFIED.,.F.,.F.,(4,1,1,1,1,1,
1,4),(91.106186954104,91.568929685544,92.5664781723222,93.5640266591005,
94.5615751458788,95.5591236326571,96.5566721194354,97.3893722612836),
 .UNSPECIFIED.);
#922=B_SPLINE_CURVE_WITH_KNOTS('',3,(#53434,#53435,#53436,#53437,#53438,
#53439,#53440,#53441,#53442,#53443,#53444),.UNSPECIFIED.,.F.,.F.,(4,1,1,
1,1,1,1,1,4),(91.106186954104,91.254149407559,92.2516978943373,93.2492463811156,
94.2467948678939,95.2443433546721,96.2418918414504,97.2394403282287,97.3893722612836),
 .UNSPECIFIED.);
#923=B_SPLINE_CURVE_WITH_KNOTS('',3,(#53449,#53450,#53451,#53452,#53453,
#53454,#53455,#53456,#53457,#53458),.UNSPECIFIED.,.F.,.F.,(4,1,1,1,1,1,
1,4),(84.8230016469244,85.5836387648743,86.5811872516526,87.5787357384309,
88.5762842252092,89.5738327119874,90.5713811987657,91.106186954104),
 .UNSPECIFIED.);
#924=B_SPLINE_CURVE_WITH_KNOTS('',3,(#53459,#53460,#53461,#53462,#53463,
#53464,#53465,#53466,#53467,#53468),.UNSPECIFIED.,.F.,.F.,(4,1,1,1,1,1,
1,4),(84.8230016469244,85.2688584868894,86.2664069736677,87.2639554604459,
88.2615039472242,89.2590524340025,90.2566009207808,91.106186954104),
 .UNSPECIFIED.);
#925=B_SPLINE_CURVE_WITH_KNOTS('',3,(#53473,#53474,#53475,#53476,#53477,
#53478,#53479,#53480,#53481,#53482,#53483),.UNSPECIFIED.,.F.,.F.,(4,1,1,
1,1,1,1,1,4),(78.5398163397448,78.6007993574264,79.5983478442047,80.595896330983,
81.5934448177612,82.5909933045395,83.5885417913178,84.5860902780961,84.8230016469244),
 .UNSPECIFIED.);
#926=B_SPLINE_CURVE_WITH_KNOTS('',3,(#53484,#53485,#53486,#53487,#53488,
#53489,#53490,#53491,#53492,#53493),.UNSPECIFIED.,.F.,.F.,(4,1,1,1,1,1,
1,4),(78.5398163397448,79.2835675662197,80.281116052998,81.2786645397763,
82.2762130265546,83.2737615133328,84.2713100001111,84.8230016469244),
 .UNSPECIFIED.);
#927=B_SPLINE_CURVE_WITH_KNOTS('',3,(#53498,#53499,#53500,#53501,#53502,
#53503,#53504,#53505,#53506,#53507),.UNSPECIFIED.,.F.,.F.,(4,1,1,1,1,1,
1,4),(72.2566310325652,72.6155084367567,73.613056923535,74.6106054103133,
75.6081538970916,76.6057023838698,77.6032508706481,78.5398163397448),
 .UNSPECIFIED.);
#928=B_SPLINE_CURVE_WITH_KNOTS('',3,(#53508,#53509,#53510,#53511,#53512,
#53513,#53514,#53515,#53516,#53517,#53518),.UNSPECIFIED.,.F.,.F.,(4,1,1,
1,1,1,1,1,4),(72.2566310325652,72.3007281587718,73.2982766455501,74.2958251323284,
75.2933736191066,76.2909221058849,77.2884705926632,78.2860190794415,78.5398163397448),
 .UNSPECIFIED.);
#929=B_SPLINE_CURVE_WITH_KNOTS('',3,(#53523,#53524,#53525,#53526,#53527,
#53528,#53529,#53530,#53531,#53532),.UNSPECIFIED.,.F.,.F.,(4,1,1,1,1,1,
1,4),(65.9734457253856,66.6302175160871,67.6277660028654,68.6253144896436,
69.6228629764219,70.6204114632002,71.6179599499785,72.2566310325652),
 .UNSPECIFIED.);
#930=B_SPLINE_CURVE_WITH_KNOTS('',3,(#53533,#53534,#53535,#53536,#53537,
#53538,#53539,#53540,#53541,#53542),.UNSPECIFIED.,.F.,.F.,(4,1,1,1,1,1,
1,4),(65.9734457253856,66.3154372381021,67.3129857248804,68.3105342116587,
69.308082698437,70.3056311852153,71.3031796719935,72.2566310325652),
 .UNSPECIFIED.);
#931=B_SPLINE_CURVE_WITH_KNOTS('',3,(#53547,#53548,#53549,#53550,#53551,
#53552,#53553,#53554,#53555,#53556),.UNSPECIFIED.,.F.,.F.,(4,1,1,1,1,1,
1,4),(59.690260418206,60.6449265954174,61.6424750821957,62.640023568974,
63.6375720557523,64.6351205425305,65.6326690293088,65.9734457253856),
 .UNSPECIFIED.);
#932=B_SPLINE_CURVE_WITH_KNOTS('',3,(#53557,#53558,#53559,#53560,#53561,
#53562,#53563,#53564,#53565,#53566),.UNSPECIFIED.,.F.,.F.,(4,1,1,1,1,1,
1,4),(59.690260418206,60.3301463174325,61.3276948042108,62.3252432909891,
63.3227917777673,64.3203402645456,65.3178887513239,65.9734457253856),
 .UNSPECIFIED.);
#933=B_SPLINE_CURVE_WITH_KNOTS('',3,(#53571,#53572,#53573,#53574,#53575,
#53576,#53577,#53578,#53579,#53580,#53581),.UNSPECIFIED.,.F.,.F.,(4,1,1,
1,1,1,1,1,4),(53.4070751110265,53.6620871879695,54.6596356747478,55.6571841615261,
56.6547326483043,57.6522811350826,58.6498296218609,59.6473781086392,59.690260418206),
 .UNSPECIFIED.);
#934=B_SPLINE_CURVE_WITH_KNOTS('',3,(#53582,#53583,#53584,#53585,#53586,
#53587,#53588,#53589,#53590,#53591),.UNSPECIFIED.,.F.,.F.,(4,1,1,1,1,1,
1,4),(53.4070751110264,54.3448553967629,55.3424038835411,56.3399523703194,
57.3375008570977,58.335049343876,59.3325978306542,59.690260418206),
 .UNSPECIFIED.);
#935=B_SPLINE_CURVE_WITH_KNOTS('',3,(#53596,#53597,#53598,#53599,#53600,
#53601,#53602,#53603,#53604,#53605),.UNSPECIFIED.,.F.,.F.,(4,1,1,1,1,1,
1,4),(47.1238898038469,47.6767962672999,48.6743447540781,49.6718932408564,
50.6694417276347,51.666990214413,52.6645387011912,53.4070751110265),
 .UNSPECIFIED.);
#936=B_SPLINE_CURVE_WITH_KNOTS('',3,(#53606,#53607,#53608,#53609,#53610,
#53611,#53612,#53613,#53614,#53615,#53616),.UNSPECIFIED.,.F.,.F.,(4,1,1,
1,1,1,1,1,4),(47.1238898038468,47.3620159893149,48.3595644760932,49.3571129628715,
50.3546614496498,51.352209936428,52.3497584232063,53.3473069099846,53.4070751110264),
 .UNSPECIFIED.);
#937=B_SPLINE_CURVE_WITH_KNOTS('',3,(#53621,#53622,#53623,#53624,#53625,
#53626,#53627,#53628,#53629,#53630),.UNSPECIFIED.,.F.,.F.,(4,1,1,1,1,1,
1,4),(40.8407044966673,41.6915053466302,42.6890538334085,43.6866023201868,
44.684150806965,45.6816992937433,46.6792477805216,47.1238898038469),
 .UNSPECIFIED.);
#938=B_SPLINE_CURVE_WITH_KNOTS('',3,(#53631,#53632,#53633,#53634,#53635,
#53636,#53637,#53638,#53639,#53640),.UNSPECIFIED.,.F.,.F.,(4,1,1,1,1,1,
1,4),(40.8407044966672,41.3767250686453,42.3742735554236,43.3718220422018,
44.3693705289801,45.3669190157584,46.3644675025367,47.1238898038468),
 .UNSPECIFIED.);
#939=B_SPLINE_CURVE_WITH_KNOTS('',3,(#53645,#53646,#53647,#53648,#53649,
#53650,#53651,#53652,#53653,#53654,#53655),.UNSPECIFIED.,.F.,.F.,(4,1,1,
1,1,1,1,1,4),(34.5575191894877,34.7086659391823,35.7062144259606,36.7037629127388,
37.7013113995171,38.6988598862954,39.6964083730737,40.6939568598519,40.8407044966673),
 .UNSPECIFIED.);
#940=B_SPLINE_CURVE_WITH_KNOTS('',3,(#53656,#53657,#53658,#53659,#53660,
#53661,#53662,#53663,#53664,#53665),.UNSPECIFIED.,.F.,.F.,(4,1,1,1,1,1,
1,4),(34.5575191894876,35.3914341479756,36.3889826347539,37.3865311215322,
38.3840796083105,39.3816280950887,40.379176581867,40.8407044966672),
 .UNSPECIFIED.);
#941=B_SPLINE_CURVE_WITH_KNOTS('',3,(#53670,#53671,#53672,#53673,#53674,
#53675,#53676,#53677,#53678,#53679),.UNSPECIFIED.,.F.,.F.,(4,1,1,1,1,1,
1,4),(28.2743338823081,28.7233750185126,29.7209235052909,30.7184719920692,
31.7160204788475,32.7135689656257,33.711117452404,34.5575191894877),
 .UNSPECIFIED.);
#942=B_SPLINE_CURVE_WITH_KNOTS('',3,(#53680,#53681,#53682,#53683,#53684,
#53685,#53686,#53687,#53688,#53689,#53690),.UNSPECIFIED.,.F.,.F.,(4,1,1,
1,1,1,1,1,4),(28.274333882308,28.4085947405277,29.406143227306,30.4036917140842,
31.4012402008625,32.3987886876408,33.3963371744191,34.3938856611974,34.5575191894876),
 .UNSPECIFIED.);
#943=B_SPLINE_CURVE_WITH_KNOTS('',3,(#53695,#53696,#53697,#53698,#53699,
#53700,#53701,#53702,#53703,#53704),.UNSPECIFIED.,.F.,.F.,(4,1,1,1,1,1,
1,4),(21.9911485751285,22.738084097843,23.7356325846212,24.7331810713995,
25.7307295581778,26.7282780449561,27.7258265317343,28.2743338823081),
 .UNSPECIFIED.);
#944=B_SPLINE_CURVE_WITH_KNOTS('',3,(#53705,#53706,#53707,#53708,#53709,
#53710,#53711,#53712,#53713,#53714),.UNSPECIFIED.,.F.,.F.,(4,1,1,1,1,1,
1,4),(21.9911485751285,22.423303819858,23.4208523066363,24.4184007934146,
25.4159492801929,26.4134977669712,27.4110462537494,28.274333882308),
 .UNSPECIFIED.);
#945=B_SPLINE_CURVE_WITH_KNOTS('',3,(#53721,#53722,#53723,#53724,#53725,
#53726,#53727,#53728,#53729,#53730),.UNSPECIFIED.,.F.,.F.,(4,1,1,1,1,1,
1,4),(15.755244690395,16.7527931771733,17.7503416639516,18.7478901507299,
19.7454386375081,20.7429871242864,21.7405356110647,21.9911485751285),
 .UNSPECIFIED.);
#946=B_SPLINE_CURVE_WITH_KNOTS('',3,(#53731,#53732,#53733,#53734,#53735,
#53736,#53737,#53738,#53739,#53740),.UNSPECIFIED.,.F.,.F.,(4,1,1,1,1,1,
1,4),(15.7079632679489,16.4380128991884,17.4355613859667,18.433109872745,
19.4306583595232,20.4282068463015,21.4257553330798,21.9911485751285),
 .UNSPECIFIED.);
#947=B_SPLINE_CURVE_WITH_KNOTS('',3,(#54166,#54167,#54168,#54169,#54170,
#54171,#54172,#54173,#54174,#54175,#54176,#54177,#54178,#54179,#54180,#54181,
#54182,#54183,#54184,#54185,#54186,#54187,#54188,#54189,#54190,#54191,#54192,
#54193,#54194,#54195,#54196,#54197,#54198,#54199,#54200,#54201,#54202,#54203,
#54204,#54205,#54206,#54207,#54208,#54209,#54210,#54211),.UNSPECIFIED.,
 .F.,.F.,(4,3,3,3,3,3,3,3,3,3,3,3,3,3,3,4),(-0.140062757837262,-0.134086502655375,
-0.12147120271553,-0.113407421882847,-0.103769248913591,-0.0940394054438087,
-0.077137461601402,-0.0675091408822671,-0.0624229504780978,-0.0526720700183036,
-0.045988001471802,-0.0296865557803863,-0.0231241453191696,-0.0164915301952035,
-0.00152741804160966,0.),.UNSPECIFIED.);
#948=B_SPLINE_CURVE_WITH_KNOTS('',3,(#54212,#54213,#54214,#54215,#54216,
#54217,#54218,#54219,#54220,#54221,#54222,#54223,#54224),.UNSPECIFIED.,
 .F.,.F.,(4,3,3,3,4),(97.5079239235673,97.759751704271,98.7573001910492,
99.7548486778275,100.674580579037),.UNSPECIFIED.);
#949=B_SPLINE_CURVE_WITH_KNOTS('',3,(#54226,#54227,#54228,#54229,#54230,
#54231,#54232,#54233,#54234,#54235,#54236,#54237,#54238,#54239,#54240,#54241,
#54242,#54243,#54244,#54245,#54246,#54247,#54248,#54249,#54250,#54251,#54252,
#54253,#54254,#54255,#54256,#54257,#54258,#54259,#54260,#54261,#54262,#54263,
#54264,#54265,#54266,#54267,#54268,#54269,#54270,#54271,#54272,#54273,#54274),
 .UNSPECIFIED.,.F.,.F.,(4,3,3,3,3,3,3,3,3,3,3,3,3,3,3,3,4),(-0.140969988491055,
-0.136418201281803,-0.126519129074011,-0.119862943924149,-0.108023198611015,
-0.101287865761346,-0.090139871551597,-0.0833947080504807,-0.0768589146704996,
-0.0729154820906274,-0.0587558950229259,-0.0520363404538416,-0.0380581629180643,
-0.0301338231072477,-0.0233108653882379,-0.00436182509706893,0.),
 .UNSPECIFIED.);
#950=B_SPLINE_CURVE_WITH_KNOTS('',3,(#54275,#54276,#54277,#54278,#54279),
 .UNSPECIFIED.,.F.,.F.,(4,1,4),(14.5207325112001,15.4404644124101,15.7079632679489),
 .UNSPECIFIED.);
#951=B_SPLINE_CURVE_WITH_KNOTS('',3,(#54281,#54282,#54283,#54284,#54285,
#54286,#54287,#54288,#54289,#54290,#54291,#54292,#54293,#54294,#54295,#54296,
#54297,#54298,#54299,#54300,#54301,#54302,#54303,#54304,#54305,#54306,#54307,
#54308,#54309,#54310,#54311,#54312,#54313,#54314,#54315,#54316,#54317,#54318,
#54319,#54320,#54321,#54322,#54323,#54324,#54325,#54326),.UNSPECIFIED.,
 .F.,.F.,(4,3,3,3,3,3,3,3,3,3,3,3,3,3,3,4),(-0.140062757837253,-0.134086502655363,
-0.121471201692539,-0.113407420189978,-0.103769238848968,-0.0940394045173825,
-0.077137458468192,-0.0675091411229651,-0.0624229504780945,-0.0526720783361747,
-0.0459880025256372,-0.0296865588875043,-0.0231241679347418,-0.0164915350738677,
-0.00152742707365775,0.),.UNSPECIFIED.);
#952=B_SPLINE_CURVE_WITH_KNOTS('',3,(#54754,#54755,#54756,#54757,#54758,
#54759,#54760,#54761,#54762,#54763,#54764,#54765,#54766,#54767,#54768,#54769,
#54770,#54771,#54772,#54773,#54774,#54775,#54776,#54777,#54778,#54779,#54780,
#54781,#54782,#54783,#54784,#54785,#54786,#54787,#54788,#54789,#54790,#54791,
#54792,#54793,#54794,#54795,#54796,#54797,#54798,#54799,#54800,#54801,#54802),
 .UNSPECIFIED.,.F.,.F.,(4,3,3,3,3,3,3,3,3,3,3,3,3,3,3,3,4),(-0.140969988491055,
-0.136418201281804,-0.12651913264835,-0.119862947097551,-0.108023216524302,
-0.101287867723297,-0.0901398753013339,-0.0833947302596222,-0.0768589166211874,
-0.0729154820906318,-0.0587558981038184,-0.0520363434544736,-0.0380581662283503,
-0.0301338238248305,-0.0233108669968244,-0.00436182790272715,0.),
 .UNSPECIFIED.);
#953=B_SPLINE_CURVE_WITH_KNOTS('',3,(#54803,#54804,#54805,#54806,#54807,
#54808,#54809,#54810,#54811,#54812),.UNSPECIFIED.,.F.,.F.,(4,3,3,4),(-102.747494138162,
-101.749945651384,-100.752397164606,-100.483683492427),.UNSPECIFIED.);
#975=SHAPE_REPRESENTATION_RELATIONSHIP('SRR','None',#55123,#995);
#995=ADVANCED_BREP_SHAPE_REPRESENTATION('',(#1035),#55001);
#1015=STYLED_ITEM('',(#55400),#1035);
#1035=MANIFOLD_SOLID_BREP('ISO_7045_M1.6x6_A2',#24548);
#1274=FACE_BOUND('',#5366,.T.);
#1275=FACE_BOUND('',#5377,.T.);
#1935=PLANE('',#27114);
#1936=PLANE('',#27119);
#1937=PLANE('',#27120);
#1938=PLANE('',#27121);
#1939=PLANE('',#27122);
#1940=PLANE('',#27123);
#1941=PLANE('',#27124);
#1942=PLANE('',#27125);
#1943=PLANE('',#27127);
#1944=PLANE('',#27128);
#1945=PLANE('',#27129);
#1946=PLANE('',#27130);
#1947=PLANE('',#27131);
#1948=PLANE('',#27132);
#1949=PLANE('',#27133);
#1950=PLANE('',#27134);
#1951=PLANE('',#27137);
#2376=CYLINDRICAL_SURFACE('',#27075,0.076925);
#2377=CYLINDRICAL_SURFACE('',#27079,0.076925);
#2378=CYLINDRICAL_SURFACE('',#27080,0.076925);
#2379=CYLINDRICAL_SURFACE('',#27081,0.076925);
#2380=CYLINDRICAL_SURFACE('',#27082,0.076925);
#2381=CYLINDRICAL_SURFACE('',#27083,0.076925);
#2382=CYLINDRICAL_SURFACE('',#27084,0.076925);
#2383=CYLINDRICAL_SURFACE('',#27085,0.076925);
#2384=CYLINDRICAL_SURFACE('',#27086,0.076925);
#2385=CYLINDRICAL_SURFACE('',#27087,0.076925);
#2386=CYLINDRICAL_SURFACE('',#27088,0.076925);
#2387=CYLINDRICAL_SURFACE('',#27089,0.076925);
#2388=CYLINDRICAL_SURFACE('',#27090,0.076925);
#2389=CYLINDRICAL_SURFACE('',#27091,0.076925);
#2390=CYLINDRICAL_SURFACE('',#27092,0.076925);
#2391=CYLINDRICAL_SURFACE('',#27093,0.076925);
#2392=CYLINDRICAL_SURFACE('',#27094,0.056925);
#2393=CYLINDRICAL_SURFACE('',#27096,0.056925);
#2394=CYLINDRICAL_SURFACE('',#27098,0.056925);
#2395=CYLINDRICAL_SURFACE('',#27099,0.056925);
#2396=CYLINDRICAL_SURFACE('',#27100,0.056925);
#2397=CYLINDRICAL_SURFACE('',#27101,0.056925);
#2398=CYLINDRICAL_SURFACE('',#27102,0.056925);
#2399=CYLINDRICAL_SURFACE('',#27103,0.056925);
#2400=CYLINDRICAL_SURFACE('',#27104,0.056925);
#2401=CYLINDRICAL_SURFACE('',#27105,0.056925);
#2402=CYLINDRICAL_SURFACE('',#27106,0.056925);
#2403=CYLINDRICAL_SURFACE('',#27107,0.056925);
#2404=CYLINDRICAL_SURFACE('',#27108,0.056925);
#2405=CYLINDRICAL_SURFACE('',#27109,0.056925);
#2406=CYLINDRICAL_SURFACE('',#27110,0.056925);
#2407=CYLINDRICAL_SURFACE('',#27111,0.056925);
#2408=CYLINDRICAL_SURFACE('',#27112,0.056925);
#2409=CYLINDRICAL_SURFACE('',#27116,0.056925);
#2410=CYLINDRICAL_SURFACE('',#27117,0.076925);
#2411=CYLINDRICAL_SURFACE('',#27139,0.16);
#3719=FACE_OUTER_BOUND('',#5321,.T.);
#3720=FACE_OUTER_BOUND('',#5322,.T.);
#3721=FACE_OUTER_BOUND('',#5323,.T.);
#3722=FACE_OUTER_BOUND('',#5324,.T.);
#3723=FACE_OUTER_BOUND('',#5325,.T.);
#3724=FACE_OUTER_BOUND('',#5326,.T.);
#3725=FACE_OUTER_BOUND('',#5327,.T.);
#3726=FACE_OUTER_BOUND('',#5328,.T.);
#3727=FACE_OUTER_BOUND('',#5329,.T.);
#3728=FACE_OUTER_BOUND('',#5330,.T.);
#3729=FACE_OUTER_BOUND('',#5331,.T.);
#3730=FACE_OUTER_BOUND('',#5332,.T.);
#3731=FACE_OUTER_BOUND('',#5333,.T.);
#3732=FACE_OUTER_BOUND('',#5334,.T.);
#3733=FACE_OUTER_BOUND('',#5335,.T.);
#3734=FACE_OUTER_BOUND('',#5336,.T.);
#3735=FACE_OUTER_BOUND('',#5337,.T.);
#3736=FACE_OUTER_BOUND('',#5338,.T.);
#3737=FACE_OUTER_BOUND('',#5339,.T.);
#3738=FACE_OUTER_BOUND('',#5340,.T.);
#3739=FACE_OUTER_BOUND('',#5341,.T.);
#3740=FACE_OUTER_BOUND('',#5342,.T.);
#3741=FACE_OUTER_BOUND('',#5343,.T.);
#3742=FACE_OUTER_BOUND('',#5344,.T.);
#3743=FACE_OUTER_BOUND('',#5345,.T.);
#3744=FACE_OUTER_BOUND('',#5346,.T.);
#3745=FACE_OUTER_BOUND('',#5347,.T.);
#3746=FACE_OUTER_BOUND('',#5348,.T.);
#3747=FACE_OUTER_BOUND('',#5349,.T.);
#3748=FACE_OUTER_BOUND('',#5350,.T.);
#3749=FACE_OUTER_BOUND('',#5351,.T.);
#3750=FACE_OUTER_BOUND('',#5352,.T.);
#3751=FACE_OUTER_BOUND('',#5353,.T.);
#3752=FACE_OUTER_BOUND('',#5354,.T.);
#3753=FACE_OUTER_BOUND('',#5355,.T.);
#3754=FACE_OUTER_BOUND('',#5356,.T.);
#3755=FACE_OUTER_BOUND('',#5357,.T.);
#3756=FACE_OUTER_BOUND('',#5358,.T.);
#3757=FACE_OUTER_BOUND('',#5359,.T.);
#3758=FACE_OUTER_BOUND('',#5360,.T.);
#3759=FACE_OUTER_BOUND('',#5361,.T.);
#3760=FACE_OUTER_BOUND('',#5362,.T.);
#3761=FACE_OUTER_BOUND('',#5363,.T.);
#3762=FACE_OUTER_BOUND('',#5364,.T.);
#3763=FACE_OUTER_BOUND('',#5365,.T.);
#3764=FACE_OUTER_BOUND('',#5367,.T.);
#3765=FACE_OUTER_BOUND('',#5368,.T.);
#3766=FACE_OUTER_BOUND('',#5369,.T.);
#3767=FACE_OUTER_BOUND('',#5370,.T.);
#3768=FACE_OUTER_BOUND('',#5371,.T.);
#3769=FACE_OUTER_BOUND('',#5372,.T.);
#3770=FACE_OUTER_BOUND('',#5373,.T.);
#3771=FACE_OUTER_BOUND('',#5374,.T.);
#3772=FACE_OUTER_BOUND('',#5375,.T.);
#3773=FACE_OUTER_BOUND('',#5376,.T.);
#3774=FACE_OUTER_BOUND('',#5378,.T.);
#3775=FACE_OUTER_BOUND('',#5379,.T.);
#5321=EDGE_LOOP('',(#22642,#22643,#22644,#22645,#22646,#22647,#22648,#22649));
#5322=EDGE_LOOP('',(#22650,#22651,#22652,#22653));
#5323=EDGE_LOOP('',(#22654,#22655,#22656,#22657));
#5324=EDGE_LOOP('',(#22658,#22659,#22660,#22661));
#5325=EDGE_LOOP('',(#22662,#22663,#22664,#22665));
#5326=EDGE_LOOP('',(#22666,#22667,#22668,#22669));
#5327=EDGE_LOOP('',(#22670,#22671,#22672,#22673));
#5328=EDGE_LOOP('',(#22674,#22675,#22676,#22677));
#5329=EDGE_LOOP('',(#22678,#22679,#22680,#22681));
#5330=EDGE_LOOP('',(#22682,#22683,#22684,#22685));
#5331=EDGE_LOOP('',(#22686,#22687,#22688,#22689));
#5332=EDGE_LOOP('',(#22690,#22691,#22692,#22693));
#5333=EDGE_LOOP('',(#22694,#22695,#22696,#22697));
#5334=EDGE_LOOP('',(#22698,#22699,#22700,#22701));
#5335=EDGE_LOOP('',(#22702,#22703,#22704,#22705));
#5336=EDGE_LOOP('',(#22706,#22707,#22708,#22709));
#5337=EDGE_LOOP('',(#22710,#22711,#22712));
#5338=EDGE_LOOP('',(#22713,#22714,#22715,#22716,#22717));
#5339=EDGE_LOOP('',(#22718,#22719,#22720,#22721));
#5340=EDGE_LOOP('',(#22722,#22723,#22724,#22725));
#5341=EDGE_LOOP('',(#22726,#22727,#22728,#22729));
#5342=EDGE_LOOP('',(#22730,#22731,#22732,#22733));
#5343=EDGE_LOOP('',(#22734,#22735,#22736,#22737));
#5344=EDGE_LOOP('',(#22738,#22739,#22740,#22741));
#5345=EDGE_LOOP('',(#22742,#22743,#22744,#22745));
#5346=EDGE_LOOP('',(#22746,#22747,#22748,#22749));
#5347=EDGE_LOOP('',(#22750,#22751,#22752,#22753));
#5348=EDGE_LOOP('',(#22754,#22755,#22756,#22757));
#5349=EDGE_LOOP('',(#22758,#22759,#22760,#22761));
#5350=EDGE_LOOP('',(#22762,#22763,#22764,#22765));
#5351=EDGE_LOOP('',(#22766,#22767,#22768,#22769));
#5352=EDGE_LOOP('',(#22770,#22771,#22772,#22773));
#5353=EDGE_LOOP('',(#22774,#22775,#22776,#22777,#22778));
#5354=EDGE_LOOP('',(#22779,#22780,#22781,#22782,#22783,#22784,#22785,#22786,
#22787,#22788,#22789,#22790,#22791,#22792,#22793,#22794,#22795,#22796,#22797,
#22798,#22799,#22800,#22801,#22802,#22803,#22804,#22805,#22806,#22807,#22808,
#22809,#22810,#22811,#22812,#22813,#22814));
#5355=EDGE_LOOP('',(#22815,#22816,#22817,#22818,#22819,#22820));
#5356=EDGE_LOOP('',(#22821,#22822,#22823));
#5357=EDGE_LOOP('',(#22824,#22825,#22826,#22827,#22828,#22829,#22830,#22831,
#22832,#22833,#22834,#22835,#22836,#22837,#22838,#22839,#22840,#22841,#22842,
#22843,#22844,#22845,#22846,#22847,#22848,#22849,#22850,#22851,#22852,#22853,
#22854,#22855,#22856,#22857,#22858,#22859));
#5358=EDGE_LOOP('',(#22860,#22861,#22862,#22863));
#5359=EDGE_LOOP('',(#22864,#22865,#22866,#22867));
#5360=EDGE_LOOP('',(#22868,#22869,#22870,#22871));
#5361=EDGE_LOOP('',(#22872,#22873,#22874,#22875));
#5362=EDGE_LOOP('',(#22876,#22877,#22878,#22879));
#5363=EDGE_LOOP('',(#22880,#22881,#22882,#22883));
#5364=EDGE_LOOP('',(#22884,#22885,#22886,#22887));
#5365=EDGE_LOOP('',(#22888));
#5366=EDGE_LOOP('',(#22889,#22890,#22891,#22892,#22893,#22894,#22895,#22896,
#22897,#22898,#22899,#22900));
#5367=EDGE_LOOP('',(#22901,#22902,#22903,#22904));
#5368=EDGE_LOOP('',(#22905,#22906,#22907,#22908));
#5369=EDGE_LOOP('',(#22909,#22910,#22911,#22912));
#5370=EDGE_LOOP('',(#22913,#22914,#22915,#22916));
#5371=EDGE_LOOP('',(#22917,#22918,#22919,#22920));
#5372=EDGE_LOOP('',(#22921,#22922,#22923,#22924));
#5373=EDGE_LOOP('',(#22925,#22926,#22927,#22928,#22929,#22930,#22931,#22932,
#22933,#22934,#22935,#22936));
#5374=EDGE_LOOP('',(#22937));
#5375=EDGE_LOOP('',(#22938,#22939,#22940,#22941));
#5376=EDGE_LOOP('',(#22942));
#5377=EDGE_LOOP('',(#22943,#22944,#22945,#22946,#22947));
#5378=EDGE_LOOP('',(#22948,#22949,#22950,#22951));
#5379=EDGE_LOOP('',(#22952,#22953,#22954,#22955));
#7128=LINE('',#52554,#8949);
#7129=LINE('',#52575,#8950);
#7130=LINE('',#52595,#8951);
#7131=LINE('',#52643,#8952);
#7132=LINE('',#52691,#8953);
#7133=LINE('',#52745,#8954);
#7134=LINE('',#52793,#8955);
#7135=LINE('',#52841,#8956);
#7136=LINE('',#52895,#8957);
#7137=LINE('',#52943,#8958);
#7138=LINE('',#52991,#8959);
#7139=LINE('',#53039,#8960);
#7140=LINE('',#53093,#8961);
#7141=LINE('',#53141,#8962);
#7142=LINE('',#53189,#8963);
#7143=LINE('',#53243,#8964);
#7144=LINE('',#53291,#8965);
#7145=LINE('',#53339,#8966);
#7146=LINE('',#53349,#8967);
#7147=LINE('',#53374,#8968);
#7148=LINE('',#53398,#8969);
#7149=LINE('',#53423,#8970);
#7150=LINE('',#53448,#8971);
#7151=LINE('',#53472,#8972);
#7152=LINE('',#53497,#8973);
#7153=LINE('',#53522,#8974);
#7154=LINE('',#53546,#8975);
#7155=LINE('',#53570,#8976);
#7156=LINE('',#53595,#8977);
#7157=LINE('',#53620,#8978);
#7158=LINE('',#53644,#8979);
#7159=LINE('',#53669,#8980);
#7160=LINE('',#53694,#8981);
#7161=LINE('',#53718,#8982);
#7162=LINE('',#54818,#8983);
#7163=LINE('',#54820,#8984);
#7164=LINE('',#54822,#8985);
#7165=LINE('',#54823,#8986);
#7166=LINE('',#54827,#8987);
#7167=LINE('',#54829,#8988);
#7168=LINE('',#54831,#8989);
#7169=LINE('',#54832,#8990);
#7170=LINE('',#54836,#8991);
#7171=LINE('',#54838,#8992);
#7172=LINE('',#54840,#8993);
#7173=LINE('',#54841,#8994);
#7174=LINE('',#54844,#8995);
#7175=LINE('',#54846,#8996);
#7176=LINE('',#54847,#8997);
#7177=LINE('',#54849,#8998);
#7178=LINE('',#54850,#8999);
#7179=LINE('',#54853,#9000);
#7180=LINE('',#54855,#9001);
#7181=LINE('',#54856,#9002);
#7182=LINE('',#54861,#9003);
#7183=LINE('',#54863,#9004);
#7184=LINE('',#54864,#9005);
#7185=LINE('',#54866,#9006);
#7186=LINE('',#54868,#9007);
#7187=LINE('',#54869,#9008);
#7188=LINE('',#54872,#9009);
#7189=LINE('',#54873,#9010);
#7190=LINE('',#54876,#9011);
#7191=LINE('',#54877,#9012);
#7192=LINE('',#54880,#9013);
#7193=LINE('',#54881,#9014);
#7194=LINE('',#54884,#9015);
#7195=LINE('',#54885,#9016);
#7196=LINE('',#54887,#9017);
#7197=LINE('',#54889,#9018);
#7198=LINE('',#54895,#9019);
#7199=LINE('',#54902,#9020);
#7200=LINE('',#54904,#9021);
#8949=VECTOR('',#33556,0.08);
#8950=VECTOR('',#33559,0.08);
#8951=VECTOR('',#33566,0.08);
#8952=VECTOR('',#33569,0.08);
#8953=VECTOR('',#33572,0.08);
#8954=VECTOR('',#33575,0.08);
#8955=VECTOR('',#33578,0.08);
#8956=VECTOR('',#33581,0.08);
#8957=VECTOR('',#33584,0.08);
#8958=VECTOR('',#33587,0.08);
#8959=VECTOR('',#33590,0.08);
#8960=VECTOR('',#33593,0.08);
#8961=VECTOR('',#33596,0.08);
#8962=VECTOR('',#33599,0.08);
#8963=VECTOR('',#33602,0.08);
#8964=VECTOR('',#33605,0.08);
#8965=VECTOR('',#33608,0.08);
#8966=VECTOR('',#33611,0.056925);
#8967=VECTOR('',#33616,0.056925);
#8968=VECTOR('',#33621,0.056925);
#8969=VECTOR('',#33624,0.056925);
#8970=VECTOR('',#33627,0.056925);
#8971=VECTOR('',#33630,0.056925);
#8972=VECTOR('',#33633,0.056925);
#8973=VECTOR('',#33636,0.056925);
#8974=VECTOR('',#33639,0.056925);
#8975=VECTOR('',#33642,0.056925);
#8976=VECTOR('',#33645,0.056925);
#8977=VECTOR('',#33648,0.056925);
#8978=VECTOR('',#33651,0.056925);
#8979=VECTOR('',#33654,0.056925);
#8980=VECTOR('',#33657,0.056925);
#8981=VECTOR('',#33660,0.056925);
#8982=VECTOR('',#33663,0.056925);
#8983=VECTOR('',#33678,1.);
#8984=VECTOR('',#33679,1.);
#8985=VECTOR('',#33680,1.);
#8986=VECTOR('',#33681,1.);
#8987=VECTOR('',#33684,1.);
#8988=VECTOR('',#33685,1.);
#8989=VECTOR('',#33686,1.);
#8990=VECTOR('',#33687,1.);
#8991=VECTOR('',#33690,1.);
#8992=VECTOR('',#33691,1.);
#8993=VECTOR('',#33692,1.);
#8994=VECTOR('',#33693,1.);
#8995=VECTOR('',#33696,1.);
#8996=VECTOR('',#33697,1.);
#8997=VECTOR('',#33698,1.);
#8998=VECTOR('',#33701,1.);
#8999=VECTOR('',#33702,1.);
#9000=VECTOR('',#33705,1.);
#9001=VECTOR('',#33706,1.);
#9002=VECTOR('',#33707,1.);
#9003=VECTOR('',#33712,1.);
#9004=VECTOR('',#33713,1.);
#9005=VECTOR('',#33714,1.);
#9006=VECTOR('',#33715,1.);
#9007=VECTOR('',#33716,1.);
#9008=VECTOR('',#33717,1.);
#9009=VECTOR('',#33720,1.);
#9010=VECTOR('',#33721,1.);
#9011=VECTOR('',#33724,1.);
#9012=VECTOR('',#33725,1.);
#9013=VECTOR('',#33728,1.);
#9014=VECTOR('',#33729,1.);
#9015=VECTOR('',#33732,1.);
#9016=VECTOR('',#33733,1.);
#9017=VECTOR('',#33736,1.);
#9018=VECTOR('',#33739,1.);
#9019=VECTOR('',#33748,0.0704);
#9020=VECTOR('',#33757,0.16);
#9021=VECTOR('',#33760,0.14375);
#10014=CIRCLE('',#27076,0.076925);
#10015=CIRCLE('',#27077,0.076925);
#10016=CIRCLE('',#27078,0.076925);
#10017=CIRCLE('',#27095,0.056925);
#10018=CIRCLE('',#27097,0.056925);
#10019=CIRCLE('',#27113,0.056925);
#10020=CIRCLE('',#27115,0.056925);
#10021=CIRCLE('',#27118,0.076925);
#10022=CIRCLE('',#27126,0.1275);
#10023=CIRCLE('',#27135,0.0608);
#10024=CIRCLE('',#27138,0.16);
#10025=CIRCLE('',#27140,0.16);
#12247=VERTEX_POINT('',#52552);
#12248=VERTEX_POINT('',#52553);
#12249=VERTEX_POINT('',#52555);
#12250=VERTEX_POINT('',#52572);
#12251=VERTEX_POINT('',#52574);
#12252=VERTEX_POINT('',#52577);
#12253=VERTEX_POINT('',#52593);
#12254=VERTEX_POINT('',#52594);
#12255=VERTEX_POINT('',#52641);
#12256=VERTEX_POINT('',#52642);
#12257=VERTEX_POINT('',#52689);
#12258=VERTEX_POINT('',#52690);
#12259=VERTEX_POINT('',#52743);
#12260=VERTEX_POINT('',#52744);
#12261=VERTEX_POINT('',#52791);
#12262=VERTEX_POINT('',#52792);
#12263=VERTEX_POINT('',#52839);
#12264=VERTEX_POINT('',#52840);
#12265=VERTEX_POINT('',#52893);
#12266=VERTEX_POINT('',#52894);
#12267=VERTEX_POINT('',#52941);
#12268=VERTEX_POINT('',#52942);
#12269=VERTEX_POINT('',#52989);
#12270=VERTEX_POINT('',#52990);
#12271=VERTEX_POINT('',#53037);
#12272=VERTEX_POINT('',#53038);
#12273=VERTEX_POINT('',#53091);
#12274=VERTEX_POINT('',#53092);
#12275=VERTEX_POINT('',#53139);
#12276=VERTEX_POINT('',#53140);
#12277=VERTEX_POINT('',#53187);
#12278=VERTEX_POINT('',#53188);
#12279=VERTEX_POINT('',#53241);
#12280=VERTEX_POINT('',#53242);
#12281=VERTEX_POINT('',#53289);
#12282=VERTEX_POINT('',#53290);
#12283=VERTEX_POINT('',#53337);
#12284=VERTEX_POINT('',#53338);
#12285=VERTEX_POINT('',#53340);
#12286=VERTEX_POINT('',#53347);
#12287=VERTEX_POINT('',#53348);
#12288=VERTEX_POINT('',#53360);
#12289=VERTEX_POINT('',#53372);
#12290=VERTEX_POINT('',#53373);
#12291=VERTEX_POINT('',#53396);
#12292=VERTEX_POINT('',#53397);
#12293=VERTEX_POINT('',#53421);
#12294=VERTEX_POINT('',#53422);
#12295=VERTEX_POINT('',#53446);
#12296=VERTEX_POINT('',#53447);
#12297=VERTEX_POINT('',#53470);
#12298=VERTEX_POINT('',#53471);
#12299=VERTEX_POINT('',#53495);
#12300=VERTEX_POINT('',#53496);
#12301=VERTEX_POINT('',#53520);
#12302=VERTEX_POINT('',#53521);
#12303=VERTEX_POINT('',#53544);
#12304=VERTEX_POINT('',#53545);
#12305=VERTEX_POINT('',#53568);
#12306=VERTEX_POINT('',#53569);
#12307=VERTEX_POINT('',#53593);
#12308=VERTEX_POINT('',#53594);
#12309=VERTEX_POINT('',#53618);
#12310=VERTEX_POINT('',#53619);
#12311=VERTEX_POINT('',#53642);
#12312=VERTEX_POINT('',#53643);
#12313=VERTEX_POINT('',#53667);
#12314=VERTEX_POINT('',#53668);
#12315=VERTEX_POINT('',#53692);
#12316=VERTEX_POINT('',#53693);
#12317=VERTEX_POINT('',#53716);
#12318=VERTEX_POINT('',#53717);
#12319=VERTEX_POINT('',#53719);
#12320=VERTEX_POINT('',#54165);
#12321=VERTEX_POINT('',#54225);
#12322=VERTEX_POINT('',#54753);
#12323=VERTEX_POINT('',#54816);
#12324=VERTEX_POINT('',#54817);
#12325=VERTEX_POINT('',#54819);
#12326=VERTEX_POINT('',#54821);
#12327=VERTEX_POINT('',#54825);
#12328=VERTEX_POINT('',#54826);
#12329=VERTEX_POINT('',#54828);
#12330=VERTEX_POINT('',#54830);
#12331=VERTEX_POINT('',#54834);
#12332=VERTEX_POINT('',#54835);
#12333=VERTEX_POINT('',#54837);
#12334=VERTEX_POINT('',#54839);
#12335=VERTEX_POINT('',#54843);
#12336=VERTEX_POINT('',#54845);
#12337=VERTEX_POINT('',#54852);
#12338=VERTEX_POINT('',#54854);
#12339=VERTEX_POINT('',#54858);
#12340=VERTEX_POINT('',#54860);
#12341=VERTEX_POINT('',#54862);
#12342=VERTEX_POINT('',#54865);
#12343=VERTEX_POINT('',#54867);
#12344=VERTEX_POINT('',#54871);
#12345=VERTEX_POINT('',#54875);
#12346=VERTEX_POINT('',#54879);
#12347=VERTEX_POINT('',#54883);
#12348=VERTEX_POINT('',#54892);
#12349=VERTEX_POINT('',#54897);
#12350=VERTEX_POINT('',#54900);
#15729=EDGE_CURVE('',#12247,#12248,#7128,.T.);
#15730=EDGE_CURVE('',#12247,#12249,#882,.T.);
#15731=EDGE_CURVE('',#12249,#12250,#10014,.T.);
#15732=EDGE_CURVE('',#12250,#12251,#7129,.T.);
#15733=EDGE_CURVE('',#12251,#12251,#10015,.T.);
#15734=EDGE_CURVE('',#12250,#12252,#10016,.T.);
#15735=EDGE_CURVE('',#12252,#12248,#883,.T.);
#15736=EDGE_CURVE('',#12253,#12254,#7130,.T.);
#15737=EDGE_CURVE('',#12253,#12247,#884,.T.);
#15738=EDGE_CURVE('',#12248,#12254,#885,.T.);
#15739=EDGE_CURVE('',#12255,#12256,#7131,.T.);
#15740=EDGE_CURVE('',#12255,#12253,#886,.T.);
#15741=EDGE_CURVE('',#12254,#12256,#887,.T.);
#15742=EDGE_CURVE('',#12257,#12258,#7132,.T.);
#15743=EDGE_CURVE('',#12257,#12255,#888,.T.);
#15744=EDGE_CURVE('',#12256,#12258,#889,.T.);
#15745=EDGE_CURVE('',#12259,#12260,#7133,.T.);
#15746=EDGE_CURVE('',#12259,#12257,#890,.T.);
#15747=EDGE_CURVE('',#12258,#12260,#891,.T.);
#15748=EDGE_CURVE('',#12261,#12262,#7134,.T.);
#15749=EDGE_CURVE('',#12261,#12259,#892,.T.);
#15750=EDGE_CURVE('',#12260,#12262,#893,.T.);
#15751=EDGE_CURVE('',#12263,#12264,#7135,.T.);
#15752=EDGE_CURVE('',#12263,#12261,#894,.T.);
#15753=EDGE_CURVE('',#12262,#12264,#895,.T.);
#15754=EDGE_CURVE('',#12265,#12266,#7136,.T.);
#15755=EDGE_CURVE('',#12265,#12263,#896,.T.);
#15756=EDGE_CURVE('',#12264,#12266,#897,.T.);
#15757=EDGE_CURVE('',#12267,#12268,#7137,.T.);
#15758=EDGE_CURVE('',#12267,#12265,#898,.T.);
#15759=EDGE_CURVE('',#12266,#12268,#899,.T.);
#15760=EDGE_CURVE('',#12269,#12270,#7138,.T.);
#15761=EDGE_CURVE('',#12269,#12267,#900,.T.);
#15762=EDGE_CURVE('',#12268,#12270,#901,.T.);
#15763=EDGE_CURVE('',#12271,#12272,#7139,.T.);
#15764=EDGE_CURVE('',#12271,#12269,#902,.T.);
#15765=EDGE_CURVE('',#12270,#12272,#903,.T.);
#15766=EDGE_CURVE('',#12273,#12274,#7140,.T.);
#15767=EDGE_CURVE('',#12273,#12271,#904,.T.);
#15768=EDGE_CURVE('',#12272,#12274,#905,.T.);
#15769=EDGE_CURVE('',#12275,#12276,#7141,.T.);
#15770=EDGE_CURVE('',#12275,#12273,#906,.T.);
#15771=EDGE_CURVE('',#12274,#12276,#907,.T.);
#15772=EDGE_CURVE('',#12277,#12278,#7142,.T.);
#15773=EDGE_CURVE('',#12277,#12275,#908,.T.);
#15774=EDGE_CURVE('',#12276,#12278,#909,.T.);
#15775=EDGE_CURVE('',#12279,#12280,#7143,.T.);
#15776=EDGE_CURVE('',#12279,#12277,#910,.T.);
#15777=EDGE_CURVE('',#12278,#12280,#911,.T.);
#15778=EDGE_CURVE('',#12281,#12282,#7144,.T.);
#15779=EDGE_CURVE('',#12281,#12279,#912,.T.);
#15780=EDGE_CURVE('',#12280,#12282,#913,.T.);
#15781=EDGE_CURVE('',#12283,#12284,#7145,.T.);
#15782=EDGE_CURVE('',#12283,#12285,#914,.T.);
#15783=EDGE_CURVE('',#12284,#12285,#10017,.T.);
#15784=EDGE_CURVE('',#12286,#12287,#7146,.T.);
#15785=EDGE_CURVE('',#12286,#12283,#915,.T.);
#15786=EDGE_CURVE('',#12288,#12284,#10018,.T.);
#15787=EDGE_CURVE('',#12287,#12288,#916,.T.);
#15788=EDGE_CURVE('',#12289,#12290,#7147,.T.);
#15789=EDGE_CURVE('',#12289,#12286,#917,.T.);
#15790=EDGE_CURVE('',#12290,#12287,#918,.T.);
#15791=EDGE_CURVE('',#12291,#12292,#7148,.T.);
#15792=EDGE_CURVE('',#12291,#12289,#919,.T.);
#15793=EDGE_CURVE('',#12292,#12290,#920,.T.);
#15794=EDGE_CURVE('',#12293,#12294,#7149,.T.);
#15795=EDGE_CURVE('',#12293,#12291,#921,.T.);
#15796=EDGE_CURVE('',#12294,#12292,#922,.T.);
#15797=EDGE_CURVE('',#12295,#12296,#7150,.T.);
#15798=EDGE_CURVE('',#12295,#12293,#923,.T.);
#15799=EDGE_CURVE('',#12296,#12294,#924,.T.);
#15800=EDGE_CURVE('',#12297,#12298,#7151,.T.);
#15801=EDGE_CURVE('',#12297,#12295,#925,.T.);
#15802=EDGE_CURVE('',#12298,#12296,#926,.T.);
#15803=EDGE_CURVE('',#12299,#12300,#7152,.T.);
#15804=EDGE_CURVE('',#12299,#12297,#927,.T.);
#15805=EDGE_CURVE('',#12300,#12298,#928,.T.);
#15806=EDGE_CURVE('',#12301,#12302,#7153,.T.);
#15807=EDGE_CURVE('',#12301,#12299,#929,.T.);
#15808=EDGE_CURVE('',#12302,#12300,#930,.T.);
#15809=EDGE_CURVE('',#12303,#12304,#7154,.T.);
#15810=EDGE_CURVE('',#12303,#12301,#931,.T.);
#15811=EDGE_CURVE('',#12304,#12302,#932,.T.);
#15812=EDGE_CURVE('',#12305,#12306,#7155,.T.);
#15813=EDGE_CURVE('',#12305,#12303,#933,.T.);
#15814=EDGE_CURVE('',#12306,#12304,#934,.T.);
#15815=EDGE_CURVE('',#12307,#12308,#7156,.T.);
#15816=EDGE_CURVE('',#12307,#12305,#935,.T.);
#15817=EDGE_CURVE('',#12308,#12306,#936,.T.);
#15818=EDGE_CURVE('',#12309,#12310,#7157,.T.);
#15819=EDGE_CURVE('',#12309,#12307,#937,.T.);
#15820=EDGE_CURVE('',#12310,#12308,#938,.T.);
#15821=EDGE_CURVE('',#12311,#12312,#7158,.T.);
#15822=EDGE_CURVE('',#12311,#12309,#939,.T.);
#15823=EDGE_CURVE('',#12312,#12310,#940,.T.);
#15824=EDGE_CURVE('',#12313,#12314,#7159,.T.);
#15825=EDGE_CURVE('',#12313,#12311,#941,.T.);
#15826=EDGE_CURVE('',#12314,#12312,#942,.T.);
#15827=EDGE_CURVE('',#12315,#12316,#7160,.T.);
#15828=EDGE_CURVE('',#12315,#12313,#943,.T.);
#15829=EDGE_CURVE('',#12316,#12314,#944,.T.);
#15830=EDGE_CURVE('',#12317,#12318,#7161,.T.);
#15831=EDGE_CURVE('',#12319,#12317,#10019,.T.);
#15832=EDGE_CURVE('',#12319,#12315,#945,.T.);
#15833=EDGE_CURVE('',#12318,#12316,#946,.T.);
#15834=EDGE_CURVE('',#12320,#12288,#947,.T.);
#15835=EDGE_CURVE('',#12282,#12320,#948,.T.);
#15836=EDGE_CURVE('',#12321,#12252,#949,.T.);
#15837=EDGE_CURVE('',#12321,#12318,#950,.T.);
#15838=EDGE_CURVE('',#12249,#12319,#951,.T.);
#15839=EDGE_CURVE('',#12317,#12321,#10020,.T.);
#15840=EDGE_CURVE('',#12285,#12322,#952,.T.);
#15841=EDGE_CURVE('',#12322,#12281,#953,.T.);
#15842=EDGE_CURVE('',#12322,#12320,#10021,.T.);
#15843=EDGE_CURVE('',#12323,#12324,#7162,.T.);
#15844=EDGE_CURVE('',#12325,#12323,#7163,.T.);
#15845=EDGE_CURVE('',#12326,#12325,#7164,.T.);
#15846=EDGE_CURVE('',#12326,#12324,#7165,.T.);
#15847=EDGE_CURVE('',#12327,#12328,#7166,.T.);
#15848=EDGE_CURVE('',#12329,#12327,#7167,.T.);
#15849=EDGE_CURVE('',#12330,#12329,#7168,.T.);
#15850=EDGE_CURVE('',#12328,#12330,#7169,.T.);
#15851=EDGE_CURVE('',#12331,#12332,#7170,.T.);
#15852=EDGE_CURVE('',#12333,#12331,#7171,.T.);
#15853=EDGE_CURVE('',#12334,#12333,#7172,.T.);
#15854=EDGE_CURVE('',#12334,#12332,#7173,.T.);
#15855=EDGE_CURVE('',#12324,#12335,#7174,.T.);
#15856=EDGE_CURVE('',#12336,#12326,#7175,.T.);
#15857=EDGE_CURVE('',#12335,#12336,#7176,.T.);
#15858=EDGE_CURVE('',#12332,#12327,#7177,.T.);
#15859=EDGE_CURVE('',#12329,#12334,#7178,.T.);
#15860=EDGE_CURVE('',#12337,#12323,#7179,.T.);
#15861=EDGE_CURVE('',#12338,#12337,#7180,.T.);
#15862=EDGE_CURVE('',#12325,#12338,#7181,.T.);
#15863=EDGE_CURVE('',#12339,#12339,#10022,.T.);
#15864=EDGE_CURVE('',#12335,#12340,#7182,.T.);
#15865=EDGE_CURVE('',#12340,#12341,#7183,.T.);
#15866=EDGE_CURVE('',#12341,#12331,#7184,.T.);
#15867=EDGE_CURVE('',#12328,#12342,#7185,.T.);
#15868=EDGE_CURVE('',#12342,#12343,#7186,.T.);
#15869=EDGE_CURVE('',#12343,#12337,#7187,.T.);
#15870=EDGE_CURVE('',#12344,#12336,#7188,.T.);
#15871=EDGE_CURVE('',#12344,#12340,#7189,.T.);
#15872=EDGE_CURVE('',#12345,#12341,#7190,.T.);
#15873=EDGE_CURVE('',#12333,#12345,#7191,.T.);
#15874=EDGE_CURVE('',#12346,#12330,#7192,.T.);
#15875=EDGE_CURVE('',#12346,#12342,#7193,.T.);
#15876=EDGE_CURVE('',#12347,#12343,#7194,.T.);
#15877=EDGE_CURVE('',#12338,#12347,#7195,.T.);
#15878=EDGE_CURVE('',#12345,#12344,#7196,.T.);
#15879=EDGE_CURVE('',#12347,#12346,#7197,.T.);
#15880=EDGE_CURVE('',#12348,#12348,#10023,.T.);
#15881=EDGE_CURVE('',#12251,#12348,#7198,.T.);
#15882=EDGE_CURVE('',#12349,#12349,#10024,.T.);
#15883=EDGE_CURVE('',#12350,#12350,#10025,.T.);
#15884=EDGE_CURVE('',#12350,#12349,#7199,.T.);
#15885=EDGE_CURVE('',#12339,#12350,#7200,.T.);
#22642=ORIENTED_EDGE('',*,*,#15729,.F.);
#22643=ORIENTED_EDGE('',*,*,#15730,.T.);
#22644=ORIENTED_EDGE('',*,*,#15731,.T.);
#22645=ORIENTED_EDGE('',*,*,#15732,.T.);
#22646=ORIENTED_EDGE('',*,*,#15733,.T.);
#22647=ORIENTED_EDGE('',*,*,#15732,.F.);
#22648=ORIENTED_EDGE('',*,*,#15734,.T.);
#22649=ORIENTED_EDGE('',*,*,#15735,.T.);
#22650=ORIENTED_EDGE('',*,*,#15736,.F.);
#22651=ORIENTED_EDGE('',*,*,#15737,.T.);
#22652=ORIENTED_EDGE('',*,*,#15729,.T.);
#22653=ORIENTED_EDGE('',*,*,#15738,.T.);
#22654=ORIENTED_EDGE('',*,*,#15739,.F.);
#22655=ORIENTED_EDGE('',*,*,#15740,.T.);
#22656=ORIENTED_EDGE('',*,*,#15736,.T.);
#22657=ORIENTED_EDGE('',*,*,#15741,.T.);
#22658=ORIENTED_EDGE('',*,*,#15742,.F.);
#22659=ORIENTED_EDGE('',*,*,#15743,.T.);
#22660=ORIENTED_EDGE('',*,*,#15739,.T.);
#22661=ORIENTED_EDGE('',*,*,#15744,.T.);
#22662=ORIENTED_EDGE('',*,*,#15745,.F.);
#22663=ORIENTED_EDGE('',*,*,#15746,.T.);
#22664=ORIENTED_EDGE('',*,*,#15742,.T.);
#22665=ORIENTED_EDGE('',*,*,#15747,.T.);
#22666=ORIENTED_EDGE('',*,*,#15748,.F.);
#22667=ORIENTED_EDGE('',*,*,#15749,.T.);
#22668=ORIENTED_EDGE('',*,*,#15745,.T.);
#22669=ORIENTED_EDGE('',*,*,#15750,.T.);
#22670=ORIENTED_EDGE('',*,*,#15751,.F.);
#22671=ORIENTED_EDGE('',*,*,#15752,.T.);
#22672=ORIENTED_EDGE('',*,*,#15748,.T.);
#22673=ORIENTED_EDGE('',*,*,#15753,.T.);
#22674=ORIENTED_EDGE('',*,*,#15754,.F.);
#22675=ORIENTED_EDGE('',*,*,#15755,.T.);
#22676=ORIENTED_EDGE('',*,*,#15751,.T.);
#22677=ORIENTED_EDGE('',*,*,#15756,.T.);
#22678=ORIENTED_EDGE('',*,*,#15757,.F.);
#22679=ORIENTED_EDGE('',*,*,#15758,.T.);
#22680=ORIENTED_EDGE('',*,*,#15754,.T.);
#22681=ORIENTED_EDGE('',*,*,#15759,.T.);
#22682=ORIENTED_EDGE('',*,*,#15760,.F.);
#22683=ORIENTED_EDGE('',*,*,#15761,.T.);
#22684=ORIENTED_EDGE('',*,*,#15757,.T.);
#22685=ORIENTED_EDGE('',*,*,#15762,.T.);
#22686=ORIENTED_EDGE('',*,*,#15763,.F.);
#22687=ORIENTED_EDGE('',*,*,#15764,.T.);
#22688=ORIENTED_EDGE('',*,*,#15760,.T.);
#22689=ORIENTED_EDGE('',*,*,#15765,.T.);
#22690=ORIENTED_EDGE('',*,*,#15766,.F.);
#22691=ORIENTED_EDGE('',*,*,#15767,.T.);
#22692=ORIENTED_EDGE('',*,*,#15763,.T.);
#22693=ORIENTED_EDGE('',*,*,#15768,.T.);
#22694=ORIENTED_EDGE('',*,*,#15769,.F.);
#22695=ORIENTED_EDGE('',*,*,#15770,.T.);
#22696=ORIENTED_EDGE('',*,*,#15766,.T.);
#22697=ORIENTED_EDGE('',*,*,#15771,.T.);
#22698=ORIENTED_EDGE('',*,*,#15772,.F.);
#22699=ORIENTED_EDGE('',*,*,#15773,.T.);
#22700=ORIENTED_EDGE('',*,*,#15769,.T.);
#22701=ORIENTED_EDGE('',*,*,#15774,.T.);
#22702=ORIENTED_EDGE('',*,*,#15775,.F.);
#22703=ORIENTED_EDGE('',*,*,#15776,.T.);
#22704=ORIENTED_EDGE('',*,*,#15772,.T.);
#22705=ORIENTED_EDGE('',*,*,#15777,.T.);
#22706=ORIENTED_EDGE('',*,*,#15778,.F.);
#22707=ORIENTED_EDGE('',*,*,#15779,.T.);
#22708=ORIENTED_EDGE('',*,*,#15775,.T.);
#22709=ORIENTED_EDGE('',*,*,#15780,.T.);
#22710=ORIENTED_EDGE('',*,*,#15781,.F.);
#22711=ORIENTED_EDGE('',*,*,#15782,.T.);
#22712=ORIENTED_EDGE('',*,*,#15783,.F.);
#22713=ORIENTED_EDGE('',*,*,#15784,.F.);
#22714=ORIENTED_EDGE('',*,*,#15785,.T.);
#22715=ORIENTED_EDGE('',*,*,#15781,.T.);
#22716=ORIENTED_EDGE('',*,*,#15786,.F.);
#22717=ORIENTED_EDGE('',*,*,#15787,.F.);
#22718=ORIENTED_EDGE('',*,*,#15788,.F.);
#22719=ORIENTED_EDGE('',*,*,#15789,.T.);
#22720=ORIENTED_EDGE('',*,*,#15784,.T.);
#22721=ORIENTED_EDGE('',*,*,#15790,.F.);
#22722=ORIENTED_EDGE('',*,*,#15791,.F.);
#22723=ORIENTED_EDGE('',*,*,#15792,.T.);
#22724=ORIENTED_EDGE('',*,*,#15788,.T.);
#22725=ORIENTED_EDGE('',*,*,#15793,.F.);
#22726=ORIENTED_EDGE('',*,*,#15794,.F.);
#22727=ORIENTED_EDGE('',*,*,#15795,.T.);
#22728=ORIENTED_EDGE('',*,*,#15791,.T.);
#22729=ORIENTED_EDGE('',*,*,#15796,.F.);
#22730=ORIENTED_EDGE('',*,*,#15797,.F.);
#22731=ORIENTED_EDGE('',*,*,#15798,.T.);
#22732=ORIENTED_EDGE('',*,*,#15794,.T.);
#22733=ORIENTED_EDGE('',*,*,#15799,.F.);
#22734=ORIENTED_EDGE('',*,*,#15800,.F.);
#22735=ORIENTED_EDGE('',*,*,#15801,.T.);
#22736=ORIENTED_EDGE('',*,*,#15797,.T.);
#22737=ORIENTED_EDGE('',*,*,#15802,.F.);
#22738=ORIENTED_EDGE('',*,*,#15803,.F.);
#22739=ORIENTED_EDGE('',*,*,#15804,.T.);
#22740=ORIENTED_EDGE('',*,*,#15800,.T.);
#22741=ORIENTED_EDGE('',*,*,#15805,.F.);
#22742=ORIENTED_EDGE('',*,*,#15806,.F.);
#22743=ORIENTED_EDGE('',*,*,#15807,.T.);
#22744=ORIENTED_EDGE('',*,*,#15803,.T.);
#22745=ORIENTED_EDGE('',*,*,#15808,.F.);
#22746=ORIENTED_EDGE('',*,*,#15809,.F.);
#22747=ORIENTED_EDGE('',*,*,#15810,.T.);
#22748=ORIENTED_EDGE('',*,*,#15806,.T.);
#22749=ORIENTED_EDGE('',*,*,#15811,.F.);
#22750=ORIENTED_EDGE('',*,*,#15812,.F.);
#22751=ORIENTED_EDGE('',*,*,#15813,.T.);
#22752=ORIENTED_EDGE('',*,*,#15809,.T.);
#22753=ORIENTED_EDGE('',*,*,#15814,.F.);
#22754=ORIENTED_EDGE('',*,*,#15815,.F.);
#22755=ORIENTED_EDGE('',*,*,#15816,.T.);
#22756=ORIENTED_EDGE('',*,*,#15812,.T.);
#22757=ORIENTED_EDGE('',*,*,#15817,.F.);
#22758=ORIENTED_EDGE('',*,*,#15818,.F.);
#22759=ORIENTED_EDGE('',*,*,#15819,.T.);
#22760=ORIENTED_EDGE('',*,*,#15815,.T.);
#22761=ORIENTED_EDGE('',*,*,#15820,.F.);
#22762=ORIENTED_EDGE('',*,*,#15821,.F.);
#22763=ORIENTED_EDGE('',*,*,#15822,.T.);
#22764=ORIENTED_EDGE('',*,*,#15818,.T.);
#22765=ORIENTED_EDGE('',*,*,#15823,.F.);
#22766=ORIENTED_EDGE('',*,*,#15824,.F.);
#22767=ORIENTED_EDGE('',*,*,#15825,.T.);
#22768=ORIENTED_EDGE('',*,*,#15821,.T.);
#22769=ORIENTED_EDGE('',*,*,#15826,.F.);
#22770=ORIENTED_EDGE('',*,*,#15827,.F.);
#22771=ORIENTED_EDGE('',*,*,#15828,.T.);
#22772=ORIENTED_EDGE('',*,*,#15824,.T.);
#22773=ORIENTED_EDGE('',*,*,#15829,.F.);
#22774=ORIENTED_EDGE('',*,*,#15830,.F.);
#22775=ORIENTED_EDGE('',*,*,#15831,.F.);
#22776=ORIENTED_EDGE('',*,*,#15832,.T.);
#22777=ORIENTED_EDGE('',*,*,#15827,.T.);
#22778=ORIENTED_EDGE('',*,*,#15833,.F.);
#22779=ORIENTED_EDGE('',*,*,#15834,.F.);
#22780=ORIENTED_EDGE('',*,*,#15835,.F.);
#22781=ORIENTED_EDGE('',*,*,#15780,.F.);
#22782=ORIENTED_EDGE('',*,*,#15777,.F.);
#22783=ORIENTED_EDGE('',*,*,#15774,.F.);
#22784=ORIENTED_EDGE('',*,*,#15771,.F.);
#22785=ORIENTED_EDGE('',*,*,#15768,.F.);
#22786=ORIENTED_EDGE('',*,*,#15765,.F.);
#22787=ORIENTED_EDGE('',*,*,#15762,.F.);
#22788=ORIENTED_EDGE('',*,*,#15759,.F.);
#22789=ORIENTED_EDGE('',*,*,#15756,.F.);
#22790=ORIENTED_EDGE('',*,*,#15753,.F.);
#22791=ORIENTED_EDGE('',*,*,#15750,.F.);
#22792=ORIENTED_EDGE('',*,*,#15747,.F.);
#22793=ORIENTED_EDGE('',*,*,#15744,.F.);
#22794=ORIENTED_EDGE('',*,*,#15741,.F.);
#22795=ORIENTED_EDGE('',*,*,#15738,.F.);
#22796=ORIENTED_EDGE('',*,*,#15735,.F.);
#22797=ORIENTED_EDGE('',*,*,#15836,.F.);
#22798=ORIENTED_EDGE('',*,*,#15837,.T.);
#22799=ORIENTED_EDGE('',*,*,#15833,.T.);
#22800=ORIENTED_EDGE('',*,*,#15829,.T.);
#22801=ORIENTED_EDGE('',*,*,#15826,.T.);
#22802=ORIENTED_EDGE('',*,*,#15823,.T.);
#22803=ORIENTED_EDGE('',*,*,#15820,.T.);
#22804=ORIENTED_EDGE('',*,*,#15817,.T.);
#22805=ORIENTED_EDGE('',*,*,#15814,.T.);
#22806=ORIENTED_EDGE('',*,*,#15811,.T.);
#22807=ORIENTED_EDGE('',*,*,#15808,.T.);
#22808=ORIENTED_EDGE('',*,*,#15805,.T.);
#22809=ORIENTED_EDGE('',*,*,#15802,.T.);
#22810=ORIENTED_EDGE('',*,*,#15799,.T.);
#22811=ORIENTED_EDGE('',*,*,#15796,.T.);
#22812=ORIENTED_EDGE('',*,*,#15793,.T.);
#22813=ORIENTED_EDGE('',*,*,#15790,.T.);
#22814=ORIENTED_EDGE('',*,*,#15787,.T.);
#22815=ORIENTED_EDGE('',*,*,#15731,.F.);
#22816=ORIENTED_EDGE('',*,*,#15838,.T.);
#22817=ORIENTED_EDGE('',*,*,#15831,.T.);
#22818=ORIENTED_EDGE('',*,*,#15839,.T.);
#22819=ORIENTED_EDGE('',*,*,#15836,.T.);
#22820=ORIENTED_EDGE('',*,*,#15734,.F.);
#22821=ORIENTED_EDGE('',*,*,#15830,.T.);
#22822=ORIENTED_EDGE('',*,*,#15837,.F.);
#22823=ORIENTED_EDGE('',*,*,#15839,.F.);
#22824=ORIENTED_EDGE('',*,*,#15840,.F.);
#22825=ORIENTED_EDGE('',*,*,#15782,.F.);
#22826=ORIENTED_EDGE('',*,*,#15785,.F.);
#22827=ORIENTED_EDGE('',*,*,#15789,.F.);
#22828=ORIENTED_EDGE('',*,*,#15792,.F.);
#22829=ORIENTED_EDGE('',*,*,#15795,.F.);
#22830=ORIENTED_EDGE('',*,*,#15798,.F.);
#22831=ORIENTED_EDGE('',*,*,#15801,.F.);
#22832=ORIENTED_EDGE('',*,*,#15804,.F.);
#22833=ORIENTED_EDGE('',*,*,#15807,.F.);
#22834=ORIENTED_EDGE('',*,*,#15810,.F.);
#22835=ORIENTED_EDGE('',*,*,#15813,.F.);
#22836=ORIENTED_EDGE('',*,*,#15816,.F.);
#22837=ORIENTED_EDGE('',*,*,#15819,.F.);
#22838=ORIENTED_EDGE('',*,*,#15822,.F.);
#22839=ORIENTED_EDGE('',*,*,#15825,.F.);
#22840=ORIENTED_EDGE('',*,*,#15828,.F.);
#22841=ORIENTED_EDGE('',*,*,#15832,.F.);
#22842=ORIENTED_EDGE('',*,*,#15838,.F.);
#22843=ORIENTED_EDGE('',*,*,#15730,.F.);
#22844=ORIENTED_EDGE('',*,*,#15737,.F.);
#22845=ORIENTED_EDGE('',*,*,#15740,.F.);
#22846=ORIENTED_EDGE('',*,*,#15743,.F.);
#22847=ORIENTED_EDGE('',*,*,#15746,.F.);
#22848=ORIENTED_EDGE('',*,*,#15749,.F.);
#22849=ORIENTED_EDGE('',*,*,#15752,.F.);
#22850=ORIENTED_EDGE('',*,*,#15755,.F.);
#22851=ORIENTED_EDGE('',*,*,#15758,.F.);
#22852=ORIENTED_EDGE('',*,*,#15761,.F.);
#22853=ORIENTED_EDGE('',*,*,#15764,.F.);
#22854=ORIENTED_EDGE('',*,*,#15767,.F.);
#22855=ORIENTED_EDGE('',*,*,#15770,.F.);
#22856=ORIENTED_EDGE('',*,*,#15773,.F.);
#22857=ORIENTED_EDGE('',*,*,#15776,.F.);
#22858=ORIENTED_EDGE('',*,*,#15779,.F.);
#22859=ORIENTED_EDGE('',*,*,#15841,.F.);
#22860=ORIENTED_EDGE('',*,*,#15778,.T.);
#22861=ORIENTED_EDGE('',*,*,#15835,.T.);
#22862=ORIENTED_EDGE('',*,*,#15842,.F.);
#22863=ORIENTED_EDGE('',*,*,#15841,.T.);
#22864=ORIENTED_EDGE('',*,*,#15843,.F.);
#22865=ORIENTED_EDGE('',*,*,#15844,.F.);
#22866=ORIENTED_EDGE('',*,*,#15845,.F.);
#22867=ORIENTED_EDGE('',*,*,#15846,.T.);
#22868=ORIENTED_EDGE('',*,*,#15847,.F.);
#22869=ORIENTED_EDGE('',*,*,#15848,.F.);
#22870=ORIENTED_EDGE('',*,*,#15849,.F.);
#22871=ORIENTED_EDGE('',*,*,#15850,.F.);
#22872=ORIENTED_EDGE('',*,*,#15851,.F.);
#22873=ORIENTED_EDGE('',*,*,#15852,.F.);
#22874=ORIENTED_EDGE('',*,*,#15853,.F.);
#22875=ORIENTED_EDGE('',*,*,#15854,.T.);
#22876=ORIENTED_EDGE('',*,*,#15855,.F.);
#22877=ORIENTED_EDGE('',*,*,#15846,.F.);
#22878=ORIENTED_EDGE('',*,*,#15856,.F.);
#22879=ORIENTED_EDGE('',*,*,#15857,.F.);
#22880=ORIENTED_EDGE('',*,*,#15858,.F.);
#22881=ORIENTED_EDGE('',*,*,#15854,.F.);
#22882=ORIENTED_EDGE('',*,*,#15859,.F.);
#22883=ORIENTED_EDGE('',*,*,#15848,.T.);
#22884=ORIENTED_EDGE('',*,*,#15860,.F.);
#22885=ORIENTED_EDGE('',*,*,#15861,.F.);
#22886=ORIENTED_EDGE('',*,*,#15862,.F.);
#22887=ORIENTED_EDGE('',*,*,#15844,.T.);
#22888=ORIENTED_EDGE('',*,*,#15863,.T.);
#22889=ORIENTED_EDGE('',*,*,#15860,.T.);
#22890=ORIENTED_EDGE('',*,*,#15843,.T.);
#22891=ORIENTED_EDGE('',*,*,#15855,.T.);
#22892=ORIENTED_EDGE('',*,*,#15864,.T.);
#22893=ORIENTED_EDGE('',*,*,#15865,.T.);
#22894=ORIENTED_EDGE('',*,*,#15866,.T.);
#22895=ORIENTED_EDGE('',*,*,#15851,.T.);
#22896=ORIENTED_EDGE('',*,*,#15858,.T.);
#22897=ORIENTED_EDGE('',*,*,#15847,.T.);
#22898=ORIENTED_EDGE('',*,*,#15867,.T.);
#22899=ORIENTED_EDGE('',*,*,#15868,.T.);
#22900=ORIENTED_EDGE('',*,*,#15869,.T.);
#22901=ORIENTED_EDGE('',*,*,#15857,.T.);
#22902=ORIENTED_EDGE('',*,*,#15870,.F.);
#22903=ORIENTED_EDGE('',*,*,#15871,.T.);
#22904=ORIENTED_EDGE('',*,*,#15864,.F.);
#22905=ORIENTED_EDGE('',*,*,#15852,.T.);
#22906=ORIENTED_EDGE('',*,*,#15866,.F.);
#22907=ORIENTED_EDGE('',*,*,#15872,.F.);
#22908=ORIENTED_EDGE('',*,*,#15873,.F.);
#22909=ORIENTED_EDGE('',*,*,#15850,.T.);
#22910=ORIENTED_EDGE('',*,*,#15874,.F.);
#22911=ORIENTED_EDGE('',*,*,#15875,.T.);
#22912=ORIENTED_EDGE('',*,*,#15867,.F.);
#22913=ORIENTED_EDGE('',*,*,#15861,.T.);
#22914=ORIENTED_EDGE('',*,*,#15869,.F.);
#22915=ORIENTED_EDGE('',*,*,#15876,.F.);
#22916=ORIENTED_EDGE('',*,*,#15877,.F.);
#22917=ORIENTED_EDGE('',*,*,#15865,.F.);
#22918=ORIENTED_EDGE('',*,*,#15871,.F.);
#22919=ORIENTED_EDGE('',*,*,#15878,.F.);
#22920=ORIENTED_EDGE('',*,*,#15872,.T.);
#22921=ORIENTED_EDGE('',*,*,#15868,.F.);
#22922=ORIENTED_EDGE('',*,*,#15875,.F.);
#22923=ORIENTED_EDGE('',*,*,#15879,.F.);
#22924=ORIENTED_EDGE('',*,*,#15876,.T.);
#22925=ORIENTED_EDGE('',*,*,#15877,.T.);
#22926=ORIENTED_EDGE('',*,*,#15879,.T.);
#22927=ORIENTED_EDGE('',*,*,#15874,.T.);
#22928=ORIENTED_EDGE('',*,*,#15849,.T.);
#22929=ORIENTED_EDGE('',*,*,#15859,.T.);
#22930=ORIENTED_EDGE('',*,*,#15853,.T.);
#22931=ORIENTED_EDGE('',*,*,#15873,.T.);
#22932=ORIENTED_EDGE('',*,*,#15878,.T.);
#22933=ORIENTED_EDGE('',*,*,#15870,.T.);
#22934=ORIENTED_EDGE('',*,*,#15856,.T.);
#22935=ORIENTED_EDGE('',*,*,#15845,.T.);
#22936=ORIENTED_EDGE('',*,*,#15862,.T.);
#22937=ORIENTED_EDGE('',*,*,#15880,.F.);
#22938=ORIENTED_EDGE('',*,*,#15733,.F.);
#22939=ORIENTED_EDGE('',*,*,#15881,.T.);
#22940=ORIENTED_EDGE('',*,*,#15880,.T.);
#22941=ORIENTED_EDGE('',*,*,#15881,.F.);
#22942=ORIENTED_EDGE('',*,*,#15882,.F.);
#22943=ORIENTED_EDGE('',*,*,#15842,.T.);
#22944=ORIENTED_EDGE('',*,*,#15834,.T.);
#22945=ORIENTED_EDGE('',*,*,#15786,.T.);
#22946=ORIENTED_EDGE('',*,*,#15783,.T.);
#22947=ORIENTED_EDGE('',*,*,#15840,.T.);
#22948=ORIENTED_EDGE('',*,*,#15883,.F.);
#22949=ORIENTED_EDGE('',*,*,#15884,.T.);
#22950=ORIENTED_EDGE('',*,*,#15882,.T.);
#22951=ORIENTED_EDGE('',*,*,#15884,.F.);
#22952=ORIENTED_EDGE('',*,*,#15863,.F.);
#22953=ORIENTED_EDGE('',*,*,#15885,.T.);
#22954=ORIENTED_EDGE('',*,*,#15883,.T.);
#22955=ORIENTED_EDGE('',*,*,#15885,.F.);
#23163=CONICAL_SURFACE('',#27136,0.0704,0.785398163397448);
#23164=CONICAL_SURFACE('',#27141,0.14375,0.558599315343562);
#24472=ADVANCED_FACE('',(#3719),#2376,.T.);
#24473=ADVANCED_FACE('',(#3720),#2377,.T.);
#24474=ADVANCED_FACE('',(#3721),#2378,.T.);
#24475=ADVANCED_FACE('',(#3722),#2379,.T.);
#24476=ADVANCED_FACE('',(#3723),#2380,.T.);
#24477=ADVANCED_FACE('',(#3724),#2381,.T.);
#24478=ADVANCED_FACE('',(#3725),#2382,.T.);
#24479=ADVANCED_FACE('',(#3726),#2383,.T.);
#24480=ADVANCED_FACE('',(#3727),#2384,.T.);
#24481=ADVANCED_FACE('',(#3728),#2385,.T.);
#24482=ADVANCED_FACE('',(#3729),#2386,.T.);
#24483=ADVANCED_FACE('',(#3730),#2387,.T.);
#24484=ADVANCED_FACE('',(#3731),#2388,.T.);
#24485=ADVANCED_FACE('',(#3732),#2389,.T.);
#24486=ADVANCED_FACE('',(#3733),#2390,.T.);
#24487=ADVANCED_FACE('',(#3734),#2391,.T.);
#24488=ADVANCED_FACE('',(#3735),#2392,.T.);
#24489=ADVANCED_FACE('',(#3736),#2393,.T.);
#24490=ADVANCED_FACE('',(#3737),#2394,.T.);
#24491=ADVANCED_FACE('',(#3738),#2395,.T.);
#24492=ADVANCED_FACE('',(#3739),#2396,.T.);
#24493=ADVANCED_FACE('',(#3740),#2397,.T.);
#24494=ADVANCED_FACE('',(#3741),#2398,.T.);
#24495=ADVANCED_FACE('',(#3742),#2399,.T.);
#24496=ADVANCED_FACE('',(#3743),#2400,.T.);
#24497=ADVANCED_FACE('',(#3744),#2401,.T.);
#24498=ADVANCED_FACE('',(#3745),#2402,.T.);
#24499=ADVANCED_FACE('',(#3746),#2403,.T.);
#24500=ADVANCED_FACE('',(#3747),#2404,.T.);
#24501=ADVANCED_FACE('',(#3748),#2405,.T.);
#24502=ADVANCED_FACE('',(#3749),#2406,.T.);
#24503=ADVANCED_FACE('',(#3750),#2407,.T.);
#24504=ADVANCED_FACE('',(#3751),#2408,.T.);
#24505=ADVANCED_FACE('',(#3752),#482,.F.);
#24506=ADVANCED_FACE('',(#3753),#1935,.T.);
#24507=ADVANCED_FACE('',(#3754),#2409,.T.);
#24508=ADVANCED_FACE('',(#3755),#483,.F.);
#24509=ADVANCED_FACE('',(#3756),#2410,.T.);
#24510=ADVANCED_FACE('',(#3757),#1936,.F.);
#24511=ADVANCED_FACE('',(#3758),#1937,.F.);
#24512=ADVANCED_FACE('',(#3759),#1938,.F.);
#24513=ADVANCED_FACE('',(#3760),#1939,.F.);
#24514=ADVANCED_FACE('',(#3761),#1940,.F.);
#24515=ADVANCED_FACE('',(#3762),#1941,.F.);
#24516=ADVANCED_FACE('',(#3763,#1274),#1942,.T.);
#24517=ADVANCED_FACE('',(#3764),#1943,.F.);
#24518=ADVANCED_FACE('',(#3765),#1944,.F.);
#24519=ADVANCED_FACE('',(#3766),#1945,.F.);
#24520=ADVANCED_FACE('',(#3767),#1946,.F.);
#24521=ADVANCED_FACE('',(#3768),#1947,.F.);
#24522=ADVANCED_FACE('',(#3769),#1948,.F.);
#24523=ADVANCED_FACE('',(#3770),#1949,.T.);
#24524=ADVANCED_FACE('',(#3771),#1950,.T.);
#24525=ADVANCED_FACE('',(#3772),#23163,.T.);
#24526=ADVANCED_FACE('',(#3773,#1275),#1951,.T.);
#24527=ADVANCED_FACE('',(#3774),#2411,.T.);
#24528=ADVANCED_FACE('',(#3775),#23164,.T.);
#24548=CLOSED_SHELL('',(#24472,#24473,#24474,#24475,#24476,#24477,#24478,
#24479,#24480,#24481,#24482,#24483,#24484,#24485,#24486,#24487,#24488,#24489,
#24490,#24491,#24492,#24493,#24494,#24495,#24496,#24497,#24498,#24499,#24500,
#24501,#24502,#24503,#24504,#24505,#24506,#24507,#24508,#24509,#24510,#24511,
#24512,#24513,#24514,#24515,#24516,#24517,#24518,#24519,#24520,#24521,#24522,
#24523,#24524,#24525,#24526,#24527,#24528));
#27074=AXIS2_PLACEMENT_3D('',#52550,#33552,#33553);
#27075=AXIS2_PLACEMENT_3D('',#52551,#33554,#33555);
#27076=AXIS2_PLACEMENT_3D('',#52573,#33557,#33558);
#27077=AXIS2_PLACEMENT_3D('',#52576,#33560,#33561);
#27078=AXIS2_PLACEMENT_3D('',#52578,#33562,#33563);
#27079=AXIS2_PLACEMENT_3D('',#52592,#33564,#33565);
#27080=AXIS2_PLACEMENT_3D('',#52640,#33567,#33568);
#27081=AXIS2_PLACEMENT_3D('',#52688,#33570,#33571);
#27082=AXIS2_PLACEMENT_3D('',#52742,#33573,#33574);
#27083=AXIS2_PLACEMENT_3D('',#52790,#33576,#33577);
#27084=AXIS2_PLACEMENT_3D('',#52838,#33579,#33580);
#27085=AXIS2_PLACEMENT_3D('',#52892,#33582,#33583);
#27086=AXIS2_PLACEMENT_3D('',#52940,#33585,#33586);
#27087=AXIS2_PLACEMENT_3D('',#52988,#33588,#33589);
#27088=AXIS2_PLACEMENT_3D('',#53036,#33591,#33592);
#27089=AXIS2_PLACEMENT_3D('',#53090,#33594,#33595);
#27090=AXIS2_PLACEMENT_3D('',#53138,#33597,#33598);
#27091=AXIS2_PLACEMENT_3D('',#53186,#33600,#33601);
#27092=AXIS2_PLACEMENT_3D('',#53240,#33603,#33604);
#27093=AXIS2_PLACEMENT_3D('',#53288,#33606,#33607);
#27094=AXIS2_PLACEMENT_3D('',#53336,#33609,#33610);
#27095=AXIS2_PLACEMENT_3D('',#53345,#33612,#33613);
#27096=AXIS2_PLACEMENT_3D('',#53346,#33614,#33615);
#27097=AXIS2_PLACEMENT_3D('',#53361,#33617,#33618);
#27098=AXIS2_PLACEMENT_3D('',#53371,#33619,#33620);
#27099=AXIS2_PLACEMENT_3D('',#53395,#33622,#33623);
#27100=AXIS2_PLACEMENT_3D('',#53420,#33625,#33626);
#27101=AXIS2_PLACEMENT_3D('',#53445,#33628,#33629);
#27102=AXIS2_PLACEMENT_3D('',#53469,#33631,#33632);
#27103=AXIS2_PLACEMENT_3D('',#53494,#33634,#33635);
#27104=AXIS2_PLACEMENT_3D('',#53519,#33637,#33638);
#27105=AXIS2_PLACEMENT_3D('',#53543,#33640,#33641);
#27106=AXIS2_PLACEMENT_3D('',#53567,#33643,#33644);
#27107=AXIS2_PLACEMENT_3D('',#53592,#33646,#33647);
#27108=AXIS2_PLACEMENT_3D('',#53617,#33649,#33650);
#27109=AXIS2_PLACEMENT_3D('',#53641,#33652,#33653);
#27110=AXIS2_PLACEMENT_3D('',#53666,#33655,#33656);
#27111=AXIS2_PLACEMENT_3D('',#53691,#33658,#33659);
#27112=AXIS2_PLACEMENT_3D('',#53715,#33661,#33662);
#27113=AXIS2_PLACEMENT_3D('',#53720,#33664,#33665);
#27114=AXIS2_PLACEMENT_3D('',#54280,#33666,#33667);
#27115=AXIS2_PLACEMENT_3D('',#54327,#33668,#33669);
#27116=AXIS2_PLACEMENT_3D('',#54328,#33670,#33671);
#27117=AXIS2_PLACEMENT_3D('',#54813,#33672,#33673);
#27118=AXIS2_PLACEMENT_3D('',#54814,#33674,#33675);
#27119=AXIS2_PLACEMENT_3D('',#54815,#33676,#33677);
#27120=AXIS2_PLACEMENT_3D('',#54824,#33682,#33683);
#27121=AXIS2_PLACEMENT_3D('',#54833,#33688,#33689);
#27122=AXIS2_PLACEMENT_3D('',#54842,#33694,#33695);
#27123=AXIS2_PLACEMENT_3D('',#54848,#33699,#33700);
#27124=AXIS2_PLACEMENT_3D('',#54851,#33703,#33704);
#27125=AXIS2_PLACEMENT_3D('',#54857,#33708,#33709);
#27126=AXIS2_PLACEMENT_3D('',#54859,#33710,#33711);
#27127=AXIS2_PLACEMENT_3D('',#54870,#33718,#33719);
#27128=AXIS2_PLACEMENT_3D('',#54874,#33722,#33723);
#27129=AXIS2_PLACEMENT_3D('',#54878,#33726,#33727);
#27130=AXIS2_PLACEMENT_3D('',#54882,#33730,#33731);
#27131=AXIS2_PLACEMENT_3D('',#54886,#33734,#33735);
#27132=AXIS2_PLACEMENT_3D('',#54888,#33737,#33738);
#27133=AXIS2_PLACEMENT_3D('',#54890,#33740,#33741);
#27134=AXIS2_PLACEMENT_3D('',#54891,#33742,#33743);
#27135=AXIS2_PLACEMENT_3D('',#54893,#33744,#33745);
#27136=AXIS2_PLACEMENT_3D('',#54894,#33746,#33747);
#27137=AXIS2_PLACEMENT_3D('',#54896,#33749,#33750);
#27138=AXIS2_PLACEMENT_3D('',#54898,#33751,#33752);
#27139=AXIS2_PLACEMENT_3D('',#54899,#33753,#33754);
#27140=AXIS2_PLACEMENT_3D('',#54901,#33755,#33756);
#27141=AXIS2_PLACEMENT_3D('',#54903,#33758,#33759);
#33552=DIRECTION('axis',(0.,0.,1.));
#33553=DIRECTION('refdir',(1.,0.,0.));
#33554=DIRECTION('center_axis',(0.,0.,1.));
#33555=DIRECTION('ref_axis',(1.,0.,0.));
#33556=DIRECTION('',(0.,0.,-1.));
#33557=DIRECTION('center_axis',(0.,0.,-1.));
#33558=DIRECTION('ref_axis',(1.,0.,0.));
#33559=DIRECTION('',(0.,0.,-1.));
#33560=DIRECTION('center_axis',(0.,0.,1.));
#33561=DIRECTION('ref_axis',(1.,0.,0.));
#33562=DIRECTION('center_axis',(0.,0.,-1.));
#33563=DIRECTION('ref_axis',(1.,0.,0.));
#33564=DIRECTION('center_axis',(0.,0.,1.));
#33565=DIRECTION('ref_axis',(1.,0.,0.));
#33566=DIRECTION('',(0.,0.,-1.));
#33567=DIRECTION('center_axis',(0.,0.,1.));
#33568=DIRECTION('ref_axis',(1.,0.,0.));
#33569=DIRECTION('',(0.,0.,-1.));
#33570=DIRECTION('center_axis',(0.,0.,1.));
#33571=DIRECTION('ref_axis',(1.,0.,0.));
#33572=DIRECTION('',(0.,0.,-1.));
#33573=DIRECTION('center_axis',(0.,0.,1.));
#33574=DIRECTION('ref_axis',(1.,0.,0.));
#33575=DIRECTION('',(0.,0.,-1.));
#33576=DIRECTION('center_axis',(0.,0.,1.));
#33577=DIRECTION('ref_axis',(1.,0.,0.));
#33578=DIRECTION('',(0.,0.,-1.));
#33579=DIRECTION('center_axis',(0.,0.,1.));
#33580=DIRECTION('ref_axis',(1.,0.,0.));
#33581=DIRECTION('',(0.,0.,-1.));
#33582=DIRECTION('center_axis',(0.,0.,1.));
#33583=DIRECTION('ref_axis',(1.,0.,0.));
#33584=DIRECTION('',(0.,0.,-1.));
#33585=DIRECTION('center_axis',(0.,0.,1.));
#33586=DIRECTION('ref_axis',(1.,0.,0.));
#33587=DIRECTION('',(0.,0.,-1.));
#33588=DIRECTION('center_axis',(0.,0.,1.));
#33589=DIRECTION('ref_axis',(1.,0.,0.));
#33590=DIRECTION('',(0.,0.,-1.));
#33591=DIRECTION('center_axis',(0.,0.,1.));
#33592=DIRECTION('ref_axis',(1.,0.,0.));
#33593=DIRECTION('',(0.,0.,-1.));
#33594=DIRECTION('center_axis',(0.,0.,1.));
#33595=DIRECTION('ref_axis',(1.,0.,0.));
#33596=DIRECTION('',(0.,0.,-1.));
#33597=DIRECTION('center_axis',(0.,0.,1.));
#33598=DIRECTION('ref_axis',(1.,0.,0.));
#33599=DIRECTION('',(0.,0.,-1.));
#33600=DIRECTION('center_axis',(0.,0.,1.));
#33601=DIRECTION('ref_axis',(1.,0.,0.));
#33602=DIRECTION('',(0.,0.,-1.));
#33603=DIRECTION('center_axis',(0.,0.,1.));
#33604=DIRECTION('ref_axis',(1.,0.,0.));
#33605=DIRECTION('',(0.,0.,-1.));
#33606=DIRECTION('center_axis',(0.,0.,1.));
#33607=DIRECTION('ref_axis',(1.,0.,0.));
#33608=DIRECTION('',(0.,0.,-1.));
#33609=DIRECTION('center_axis',(0.,0.,1.));
#33610=DIRECTION('ref_axis',(1.,1.10752194731043E-13,0.));
#33611=DIRECTION('',(0.,0.,1.));
#33612=DIRECTION('center_axis',(0.,0.,1.));
#33613=DIRECTION('ref_axis',(1.,1.10752194731043E-13,0.));
#33614=DIRECTION('center_axis',(0.,0.,1.));
#33615=DIRECTION('ref_axis',(1.,1.10752194731043E-13,0.));
#33616=DIRECTION('',(0.,0.,1.));
#33617=DIRECTION('center_axis',(0.,0.,1.));
#33618=DIRECTION('ref_axis',(1.,1.10752194731043E-13,0.));
#33619=DIRECTION('center_axis',(0.,0.,1.));
#33620=DIRECTION('ref_axis',(1.,1.10752194731043E-13,0.));
#33621=DIRECTION('',(0.,0.,1.));
#33622=DIRECTION('center_axis',(0.,0.,1.));
#33623=DIRECTION('ref_axis',(1.,1.10752194731043E-13,0.));
#33624=DIRECTION('',(0.,0.,1.));
#33625=DIRECTION('center_axis',(0.,0.,1.));
#33626=DIRECTION('ref_axis',(1.,1.10752194731043E-13,0.));
#33627=DIRECTION('',(0.,0.,1.));
#33628=DIRECTION('center_axis',(0.,0.,1.));
#33629=DIRECTION('ref_axis',(1.,1.10752194731043E-13,0.));
#33630=DIRECTION('',(0.,0.,1.));
#33631=DIRECTION('center_axis',(0.,0.,1.));
#33632=DIRECTION('ref_axis',(1.,1.10752194731043E-13,0.));
#33633=DIRECTION('',(0.,0.,1.));
#33634=DIRECTION('center_axis',(0.,0.,1.));
#33635=DIRECTION('ref_axis',(1.,1.10752194731043E-13,0.));
#33636=DIRECTION('',(0.,0.,1.));
#33637=DIRECTION('center_axis',(0.,0.,1.));
#33638=DIRECTION('ref_axis',(1.,1.10752194731043E-13,0.));
#33639=DIRECTION('',(0.,0.,1.));
#33640=DIRECTION('center_axis',(0.,0.,1.));
#33641=DIRECTION('ref_axis',(1.,1.10752194731043E-13,0.));
#33642=DIRECTION('',(0.,0.,1.));
#33643=DIRECTION('center_axis',(0.,0.,1.));
#33644=DIRECTION('ref_axis',(1.,1.10752194731043E-13,0.));
#33645=DIRECTION('',(0.,0.,1.));
#33646=DIRECTION('center_axis',(0.,0.,1.));
#33647=DIRECTION('ref_axis',(1.,1.10752194731043E-13,0.));
#33648=DIRECTION('',(0.,0.,1.));
#33649=DIRECTION('center_axis',(0.,0.,1.));
#33650=DIRECTION('ref_axis',(1.,1.10752194731043E-13,0.));
#33651=DIRECTION('',(0.,0.,1.));
#33652=DIRECTION('center_axis',(0.,0.,1.));
#33653=DIRECTION('ref_axis',(1.,1.10752194731043E-13,0.));
#33654=DIRECTION('',(0.,0.,1.));
#33655=DIRECTION('center_axis',(0.,0.,1.));
#33656=DIRECTION('ref_axis',(1.,1.10752194731043E-13,0.));
#33657=DIRECTION('',(0.,0.,1.));
#33658=DIRECTION('center_axis',(0.,0.,1.));
#33659=DIRECTION('ref_axis',(1.,1.10752194731043E-13,0.));
#33660=DIRECTION('',(0.,0.,1.));
#33661=DIRECTION('center_axis',(0.,0.,1.));
#33662=DIRECTION('ref_axis',(1.,1.10752194731043E-13,0.));
#33663=DIRECTION('',(0.,0.,1.));
#33664=DIRECTION('center_axis',(0.,0.,-1.));
#33665=DIRECTION('ref_axis',(1.,1.10752194731043E-13,0.));
#33666=DIRECTION('center_axis',(0.,0.,1.));
#33667=DIRECTION('ref_axis',(1.,0.,0.));
#33668=DIRECTION('center_axis',(0.,0.,-1.));
#33669=DIRECTION('ref_axis',(1.,1.10752194731043E-13,0.));
#33670=DIRECTION('center_axis',(0.,0.,1.));
#33671=DIRECTION('ref_axis',(1.,1.10752194731043E-13,0.));
#33672=DIRECTION('center_axis',(0.,0.,1.));
#33673=DIRECTION('ref_axis',(1.,0.,0.));
#33674=DIRECTION('center_axis',(0.,0.,1.));
#33675=DIRECTION('ref_axis',(1.,0.,0.));
#33676=DIRECTION('center_axis',(0.,-1.,0.));
#33677=DIRECTION('ref_axis',(1.,0.,0.));
#33678=DIRECTION('',(-1.,0.,0.));
#33679=DIRECTION('',(0.,0.,1.));
#33680=DIRECTION('',(1.,0.,0.));
#33681=DIRECTION('',(0.,0.,1.));
#33682=DIRECTION('center_axis',(1.,0.,0.));
#33683=DIRECTION('ref_axis',(0.,1.,0.));
#33684=DIRECTION('',(0.,-1.,0.));
#33685=DIRECTION('',(0.,0.,1.));
#33686=DIRECTION('',(0.,1.,0.));
#33687=DIRECTION('',(0.,0.,-1.));
#33688=DIRECTION('center_axis',(-1.,0.,0.));
#33689=DIRECTION('ref_axis',(0.,-1.,0.));
#33690=DIRECTION('',(0.,1.,0.));
#33691=DIRECTION('',(0.,0.,1.));
#33692=DIRECTION('',(0.,-1.,0.));
#33693=DIRECTION('',(0.,0.,1.));
#33694=DIRECTION('center_axis',(-1.,0.,0.));
#33695=DIRECTION('ref_axis',(0.,-1.,0.));
#33696=DIRECTION('',(0.,1.,0.));
#33697=DIRECTION('',(0.,-1.,0.));
#33698=DIRECTION('',(0.,0.,-1.));
#33699=DIRECTION('center_axis',(0.,1.,0.));
#33700=DIRECTION('ref_axis',(-1.,0.,0.));
#33701=DIRECTION('',(1.,0.,0.));
#33702=DIRECTION('',(-1.,0.,0.));
#33703=DIRECTION('center_axis',(1.,0.,0.));
#33704=DIRECTION('ref_axis',(0.,1.,0.));
#33705=DIRECTION('',(0.,-1.,0.));
#33706=DIRECTION('',(0.,0.,1.));
#33707=DIRECTION('',(0.,1.,0.));
#33708=DIRECTION('center_axis',(0.,0.,1.));
#33709=DIRECTION('ref_axis',(1.,0.,0.));
#33710=DIRECTION('center_axis',(0.,0.,1.));
#33711=DIRECTION('ref_axis',(1.,0.,0.));
#33712=DIRECTION('',(-1.,0.,0.));
#33713=DIRECTION('',(0.,1.,0.));
#33714=DIRECTION('',(1.,0.,0.));
#33715=DIRECTION('',(1.,0.,0.));
#33716=DIRECTION('',(0.,-1.,0.));
#33717=DIRECTION('',(-1.,0.,0.));
#33718=DIRECTION('center_axis',(0.,-1.,0.));
#33719=DIRECTION('ref_axis',(1.,0.,0.));
#33720=DIRECTION('',(1.,0.,0.));
#33721=DIRECTION('',(0.,0.,1.));
#33722=DIRECTION('center_axis',(0.,1.,0.));
#33723=DIRECTION('ref_axis',(-1.,0.,0.));
#33724=DIRECTION('',(0.,0.,1.));
#33725=DIRECTION('',(-1.,0.,0.));
#33726=DIRECTION('center_axis',(0.,1.,0.));
#33727=DIRECTION('ref_axis',(-1.,0.,0.));
#33728=DIRECTION('',(-1.,0.,0.));
#33729=DIRECTION('',(0.,0.,1.));
#33730=DIRECTION('center_axis',(0.,-1.,0.));
#33731=DIRECTION('ref_axis',(1.,0.,0.));
#33732=DIRECTION('',(0.,0.,1.));
#33733=DIRECTION('',(1.,0.,0.));
#33734=DIRECTION('center_axis',(-1.,0.,0.));
#33735=DIRECTION('ref_axis',(0.,-1.,0.));
#33736=DIRECTION('',(0.,-1.,0.));
#33737=DIRECTION('center_axis',(1.,0.,0.));
#33738=DIRECTION('ref_axis',(0.,1.,0.));
#33739=DIRECTION('',(0.,1.,0.));
#33740=DIRECTION('center_axis',(0.,0.,1.));
#33741=DIRECTION('ref_axis',(1.,0.,0.));
#33742=DIRECTION('center_axis',(0.,0.,-1.));
#33743=DIRECTION('ref_axis',(-1.,0.,0.));
#33744=DIRECTION('center_axis',(0.,0.,1.));
#33745=DIRECTION('ref_axis',(1.,0.,0.));
#33746=DIRECTION('center_axis',(0.,0.,1.));
#33747=DIRECTION('ref_axis',(1.,0.,0.));
#33748=DIRECTION('',(0.707106781186548,8.65956056235493E-17,-0.707106781186548));
#33749=DIRECTION('center_axis',(0.,0.,-1.));
#33750=DIRECTION('ref_axis',(-1.,0.,0.));
#33751=DIRECTION('center_axis',(0.,0.,1.));
#33752=DIRECTION('ref_axis',(1.,0.,0.));
#33753=DIRECTION('center_axis',(0.,0.,1.));
#33754=DIRECTION('ref_axis',(1.,0.,0.));
#33755=DIRECTION('center_axis',(0.,0.,1.));
#33756=DIRECTION('ref_axis',(1.,0.,0.));
#33757=DIRECTION('',(0.,0.,-1.));
#33758=DIRECTION('center_axis',(0.,0.,-1.));
#33759=DIRECTION('ref_axis',(1.,0.,0.));
#33760=DIRECTION('',(-0.52999894000318,-6.49061505426384E-17,-0.847998304005088));
#52550=CARTESIAN_POINT('',(0.,0.,0.));
#52551=CARTESIAN_POINT('Origin',(0.,0.,-0.2904));
#52552=CARTESIAN_POINT('',(-0.0769096047044028,6.91658437555233E-5,-0.537610382907248));
#52553=CARTESIAN_POINT('',(-0.0768915057166184,6.11931288171008E-5,-0.542639617092752));
#52554=CARTESIAN_POINT('',(-0.076925,-9.42059550244101E-18,-0.2904));
#52555=CARTESIAN_POINT('',(0.040207606550226,-0.0657262044767398,-0.5608));
#52556=CARTESIAN_POINT('Ctrl Pts',(-0.0769096047044028,6.91658437555233E-5,
-0.537610382907248));
#52557=CARTESIAN_POINT('Ctrl Pts',(-0.0769675453873495,0.00649632637372731,
-0.538075722980974));
#52558=CARTESIAN_POINT('Ctrl Pts',(-0.0762292291219459,0.012910442097877,
-0.5385410630547));
#52559=CARTESIAN_POINT('Ctrl Pts',(-0.0746430427302316,0.019107617912474,
-0.539006403128426));
#52560=CARTESIAN_POINT('Ctrl Pts',(-0.0683293317028954,0.0437750702896657,
-0.54085865880928));
#52561=CARTESIAN_POINT('Ctrl Pts',(-0.0485820861472687,0.0650053573804454,
-0.542710914490134));
#52562=CARTESIAN_POINT('Ctrl Pts',(-0.0244321386735508,0.0730771079271841,
-0.544563170170987));
#52563=CARTESIAN_POINT('Ctrl Pts',(-0.000282191199832891,0.0811488584739228,
-0.546415425851841));
#52564=CARTESIAN_POINT('Ctrl Pts',(0.0282704581919762,0.0760620724766204,
-0.548267681532694));
#52565=CARTESIAN_POINT('Ctrl Pts',(0.0481472482356463,0.0601553154154528,
-0.550119937213548));
#52566=CARTESIAN_POINT('Ctrl Pts',(0.0680240382793164,0.0442485583542852,
-0.551972192894402));
#52567=CARTESIAN_POINT('Ctrl Pts',(0.0792249689748476,0.0175218302292525,
-0.553824448575256));
#52568=CARTESIAN_POINT('Ctrl Pts',(0.0766467092357258,-0.0078140970938064,
-0.55567670425611));
#52569=CARTESIAN_POINT('Ctrl Pts',(0.0742695739254072,-0.031173623888351,
-0.557384469504073));
#52570=CARTESIAN_POINT('Ctrl Pts',(0.0601791680603887,-0.0533508732364468,
-0.559092234752036));
#52571=CARTESIAN_POINT('Ctrl Pts',(0.040207606550226,-0.0657262044767398,
-0.5608));
#52572=CARTESIAN_POINT('',(-0.076925,-9.42059550244101E-18,-0.5608));
#52573=CARTESIAN_POINT('Origin',(0.,0.,-0.5608));
#52574=CARTESIAN_POINT('',(-0.076925,-9.42059550244101E-18,-0.583875));
#52575=CARTESIAN_POINT('',(-0.076925,-9.42059550244101E-18,-0.2904));
#52576=CARTESIAN_POINT('Origin',(0.,0.,-0.583875));
#52577=CARTESIAN_POINT('',(0.076385061748025,-0.00909823976109752,-0.5608));
#52578=CARTESIAN_POINT('Origin',(0.,0.,-0.5608));
#52579=CARTESIAN_POINT('Ctrl Pts',(0.0763850617480249,-0.00909823976109754,
-0.5608));
#52580=CARTESIAN_POINT('Ctrl Pts',(0.079410373516701,0.0163010278253042,
-0.558947744319146));
#52581=CARTESIAN_POINT('Ctrl Pts',(0.0687474789230948,0.0431078601247894,
-0.557095488638293));
#52582=CARTESIAN_POINT('Ctrl Pts',(0.0491671677694739,0.0593179775882079,
-0.555243232957439));
#52583=CARTESIAN_POINT('Ctrl Pts',(0.0295868566158525,0.0755280950516269,
-0.553390977276585));
#52584=CARTESIAN_POINT('Ctrl Pts',(0.00108912890221588,0.0811414976789785,
-0.551538721595731));
#52585=CARTESIAN_POINT('Ctrl Pts',(-0.0232026118821274,0.0734899793472007,
-0.549686465914878));
#52586=CARTESIAN_POINT('Ctrl Pts',(-0.0474943526664708,0.065838461015423,
-0.547834210234024));
#52587=CARTESIAN_POINT('Ctrl Pts',(-0.0675801065215208,0.0449220217245157,
-0.54598195455317));
#52588=CARTESIAN_POINT('Ctrl Pts',(-0.0743052974197677,0.0203592775072516,
-0.544129698872317));
#52589=CARTESIAN_POINT('Ctrl Pts',(-0.0761086993520085,0.0137726242727538,
-0.543633004945795));
#52590=CARTESIAN_POINT('Ctrl Pts',(-0.076951372979264,0.006923773377672,
-0.543136311019274));
#52591=CARTESIAN_POINT('Ctrl Pts',(-0.0768915057166184,6.11931288171008E-5,
-0.542639617092752));
#52592=CARTESIAN_POINT('Origin',(0.,0.,-0.2904));
#52593=CARTESIAN_POINT('',(-0.0768038780644556,-2.07208059154612E-5,-0.502610382907248));
#52594=CARTESIAN_POINT('',(-0.0768078911416689,-2.75047320366774E-5,-0.507639617092753));
#52595=CARTESIAN_POINT('',(-0.076925,-9.42059550244101E-18,-0.2904));
#52596=CARTESIAN_POINT('Ctrl Pts',(-0.0768038780644556,-2.07208059154612E-5,
-0.502610382907248));
#52597=CARTESIAN_POINT('Ctrl Pts',(-0.0767698356268339,0.0140956948725698,
-0.503628855562518));
#52598=CARTESIAN_POINT('Ctrl Pts',(-0.0730479576749677,0.0282288086778181,
-0.504647328217789));
#52599=CARTESIAN_POINT('Ctrl Pts',(-0.0657479191161002,0.0401754805758868,
-0.50566580087306));
#52600=CARTESIAN_POINT('Ctrl Pts',(-0.0524716295454961,0.0619024172550219,
-0.507518056553913));
#52601=CARTESIAN_POINT('Ctrl Pts',(-0.0273604846150267,0.0763976428495325,
-0.509370312234767));
#52602=CARTESIAN_POINT('Ctrl Pts',(-0.00190612534401761,0.0770274929451187,
-0.511222567915621));
#52603=CARTESIAN_POINT('Ctrl Pts',(0.0235482339269917,0.0776573430407048,
-0.513074823596474));
#52604=CARTESIAN_POINT('Ctrl Pts',(0.0493458075385404,0.0644218176373664,
-0.514927079277328));
#52605=CARTESIAN_POINT('Ctrl Pts',(0.0636804316029636,0.0433782047807641,
-0.516779334958182));
#52606=CARTESIAN_POINT('Ctrl Pts',(0.0780150556673868,0.0223345919241618,
-0.518631590639035));
#52607=CARTESIAN_POINT('Ctrl Pts',(0.080886730184684,-0.00651710838570469,
-0.520483846319889));
#52608=CARTESIAN_POINT('Ctrl Pts',(0.0709817539352405,-0.0299737413516422,
-0.522336102000743));
#52609=CARTESIAN_POINT('Ctrl Pts',(0.0610767776857971,-0.0534303743175797,
-0.524188357681596));
#52610=CARTESIAN_POINT('Ctrl Pts',(0.0383951506696132,-0.0714919399395886,
-0.52604061336245));
#52611=CARTESIAN_POINT('Ctrl Pts',(0.0133158987600065,-0.0758919834556476,
-0.527892869043304));
#52612=CARTESIAN_POINT('Ctrl Pts',(-0.0117633531496002,-0.0802920269717066,
-0.529745124724158));
#52613=CARTESIAN_POINT('Ctrl Pts',(-0.0392402299526296,-0.0710305483818158,
-0.531597380405011));
#52614=CARTESIAN_POINT('Ctrl Pts',(-0.0565385801046214,-0.0523475002550685,
-0.533449636085865));
#52615=CARTESIAN_POINT('Ctrl Pts',(-0.069491085555866,-0.038358172915681,
-0.534836551692993));
#52616=CARTESIAN_POINT('Ctrl Pts',(-0.0767369162943482,-0.0190865650976122,
-0.53622346730012));
#52617=CARTESIAN_POINT('Ctrl Pts',(-0.0769096047044028,6.91658437555233E-5,
-0.537610382907248));
#52618=CARTESIAN_POINT('Ctrl Pts',(-0.0768915057166184,6.11931288171008E-5,
-0.542639617092752));
#52619=CARTESIAN_POINT('Ctrl Pts',(-0.0767281178287347,-0.0186679493564494,
-0.54128405533842));
#52620=CARTESIAN_POINT('Ctrl Pts',(-0.0698422765132579,-0.037499353071499,
-0.539928493584088));
#52621=CARTESIAN_POINT('Ctrl Pts',(-0.0574168066131572,-0.0513821924115064,
-0.538572931829756));
#52622=CARTESIAN_POINT('Ctrl Pts',(-0.0404384969668562,-0.0703518689693793,
-0.536720676148902));
#52623=CARTESIAN_POINT('Ctrl Pts',(-0.0131172497328104,-0.0800821729415043,
-0.534868420468049));
#52624=CARTESIAN_POINT('Ctrl Pts',(0.0120338256236662,-0.0761076871249378,
-0.533016164787195));
#52625=CARTESIAN_POINT('Ctrl Pts',(0.0371849009801429,-0.0721332013083712,
-0.531163909106341));
#52626=CARTESIAN_POINT('Ctrl Pts',(0.0601658044590504,-0.0544539257031128,
-0.529311653425487));
#52627=CARTESIAN_POINT('Ctrl Pts',(0.0704648543013367,-0.0311671118066004,
-0.527459397744633));
#52628=CARTESIAN_POINT('Ctrl Pts',(0.080763904143623,-0.00788029791008813,
-0.525607142063779));
#52629=CARTESIAN_POINT('Ctrl Pts',(0.0783811003492882,0.0210140542776783,
-0.523754886382926));
#52630=CARTESIAN_POINT('Ctrl Pts',(0.0644041500243277,0.042296301050223,
-0.521902630702073));
#52631=CARTESIAN_POINT('Ctrl Pts',(0.0504271996993672,0.0635785478227678,
-0.520050375021219));
#52632=CARTESIAN_POINT('Ctrl Pts',(0.024856102843781,0.077248689180091,
-0.518198119340365));
#52633=CARTESIAN_POINT('Ctrl Pts',(-0.000605423883035404,0.0770489427047095,
-0.516345863659511));
#52634=CARTESIAN_POINT('Ctrl Pts',(-0.0260669506098518,0.0768491962293279,
-0.514493607978657));
#52635=CARTESIAN_POINT('Ctrl Pts',(-0.0514189072078984,0.0627795619212417,
-0.512641352297804));
#52636=CARTESIAN_POINT('Ctrl Pts',(-0.0650600797594811,0.0412797811922074,
-0.51078909661695));
#52637=CARTESIAN_POINT('Ctrl Pts',(-0.0727916606064359,0.0290940770476583,
-0.509739270108885));
#52638=CARTESIAN_POINT('Ctrl Pts',(-0.0767612381677875,0.0145214929865115,
-0.508689443600819));
#52639=CARTESIAN_POINT('Ctrl Pts',(-0.0768078911416689,-2.75047320366774E-5,
-0.507639617092753));
#52640=CARTESIAN_POINT('Origin',(0.,0.,-0.2904));
#52641=CARTESIAN_POINT('',(-0.0769866657903101,-5.93158920058345E-5,-0.467610382907248));
#52642=CARTESIAN_POINT('',(-0.0769983882791968,-5.48405244063995E-5,-0.472639617092753));
#52643=CARTESIAN_POINT('',(-0.076925,-9.42059550244101E-18,-0.2904));
#52644=CARTESIAN_POINT('Ctrl Pts',(-0.0769866657903101,-5.93158920058345E-5,
-0.467610382907248));
#52645=CARTESIAN_POINT('Ctrl Pts',(-0.0768022090703362,0.0215924718018981,
-0.469181988144063));
#52646=CARTESIAN_POINT('Ctrl Pts',(-0.0672397070232822,0.0433868987541688,
-0.470753593380878));
#52647=CARTESIAN_POINT('Ctrl Pts',(-0.0510603483059523,0.0577035795188773,
-0.472325198617693));
#52648=CARTESIAN_POINT('Ctrl Pts',(-0.0319917499106721,0.0745768710148652,
-0.474177454298547));
#52649=CARTESIAN_POINT('Ctrl Pts',(-0.00373206903032697,0.0810632695438336,
-0.4760297099794));
#52650=CARTESIAN_POINT('Ctrl Pts',(0.0207860373958043,0.0741943601536088,
-0.477881965660254));
#52651=CARTESIAN_POINT('Ctrl Pts',(0.0453041438219356,0.067325450763384,
-0.479734221341108));
#52652=CARTESIAN_POINT('Ctrl Pts',(0.066080675793853,0.0471012334539661,
-0.481586477021962));
#52653=CARTESIAN_POINT('Ctrl Pts',(0.0736075296600365,0.0227770520257243,
-0.483438732702815));
#52654=CARTESIAN_POINT('Ctrl Pts',(0.08113438352622,-0.00154712940251749,
-0.485290988383669));
#52655=CARTESIAN_POINT('Ctrl Pts',(0.0754115592866696,-0.0299712749495833,
-0.487143244064522));
#52656=CARTESIAN_POINT('Ctrl Pts',(0.0590580402410755,-0.0494874691264555,
-0.488995499745376));
#52657=CARTESIAN_POINT('Ctrl Pts',(0.0427045211954813,-0.069003663303328,
-0.49084775542623));
#52658=CARTESIAN_POINT('Ctrl Pts',(0.0157203073438432,-0.0796119061100067,
-0.492700011107084));
#52659=CARTESIAN_POINT('Ctrl Pts',(-0.00954566134870712,-0.0764574612990264,
-0.494552266787938));
#52660=CARTESIAN_POINT('Ctrl Pts',(-0.0348116300412571,-0.0733030164880461,
-0.496404522468791));
#52661=CARTESIAN_POINT('Ctrl Pts',(-0.0583593535747193,-0.0563858840594071,
-0.498256778149645));
#52662=CARTESIAN_POINT('Ctrl Pts',(-0.0694124982360811,-0.0334479939632078,
-0.500109033830498));
#52663=CARTESIAN_POINT('Ctrl Pts',(-0.0743880124122404,-0.0231226249536286,
-0.500942816856081));
#52664=CARTESIAN_POINT('Ctrl Pts',(-0.0768317472531782,-0.0115772684597858,
-0.501776599881665));
#52665=CARTESIAN_POINT('Ctrl Pts',(-0.0768038780644556,-2.07208059154612E-5,
-0.502610382907248));
#52666=CARTESIAN_POINT('Ctrl Pts',(-0.0768078911416689,-2.75047320366774E-5,
-0.507639617092753));
#52667=CARTESIAN_POINT('Ctrl Pts',(-0.0768435500881255,-0.0111479518863914,
-0.506837187919965));
#52668=CARTESIAN_POINT('Ctrl Pts',(-0.0745873478507643,-0.0222546193664585,
-0.506034758747177));
#52669=CARTESIAN_POINT('Ctrl Pts',(-0.0699674254473345,-0.0322711198318006,
-0.505232329574389));
#52670=CARTESIAN_POINT('Ctrl Pts',(-0.0593032100784864,-0.0553923129767922,
-0.503380073893535));
#52671=CARTESIAN_POINT('Ctrl Pts',(-0.0360443908356715,-0.0727047721167927,
-0.501527818212681));
#52672=CARTESIAN_POINT('Ctrl Pts',(-0.0108352639658483,-0.0762854167965552,
-0.499675562531828));
#52673=CARTESIAN_POINT('Ctrl Pts',(0.0143738629039748,-0.0798660614763177,
-0.497823306850974));
#52674=CARTESIAN_POINT('Ctrl Pts',(0.0415332974008062,-0.0697148916958422,
-0.495971051170121));
#52675=CARTESIAN_POINT('Ctrl Pts',(0.0582140048717536,-0.0504775941790726,
-0.494118795489267));
#52676=CARTESIAN_POINT('Ctrl Pts',(0.0748947123427012,-0.0312402966623029,
-0.492266539808413));
#52677=CARTESIAN_POINT('Ctrl Pts',(0.0810966927877647,-0.00291687140923884,
-0.490414284127559));
#52678=CARTESIAN_POINT('Ctrl Pts',(0.0739816346844856,0.0215309246469676,
-0.488562028446706));
#52679=CARTESIAN_POINT('Ctrl Pts',(0.0668665765812064,0.045978720703174,
-0.486709772765852));
#52680=CARTESIAN_POINT('Ctrl Pts',(0.0464344799295845,0.0665508875625229,
-0.484857517084999));
#52681=CARTESIAN_POINT('Ctrl Pts',(0.0220358480118087,0.0738328125955258,
-0.483005261404145));
#52682=CARTESIAN_POINT('Ctrl Pts',(-0.00236278390596698,0.0811147376285286,
-0.481153005723291));
#52683=CARTESIAN_POINT('Ctrl Pts',(-0.0307279510898964,0.0751064208351859,
-0.479300750042437));
#52684=CARTESIAN_POINT('Ctrl Pts',(-0.0500787358259481,0.058557507707521,
-0.477448494361583));
#52685=CARTESIAN_POINT('Ctrl Pts',(-0.0668250827824603,0.0442359261918763,
-0.475845535271973));
#52686=CARTESIAN_POINT('Ctrl Pts',(-0.0768202606431028,0.0220201435331388,
-0.474242576182363));
#52687=CARTESIAN_POINT('Ctrl Pts',(-0.0769983882791968,-5.48405244063995E-5,
-0.472639617092753));
#52688=CARTESIAN_POINT('Origin',(0.,0.,-0.2904));
#52689=CARTESIAN_POINT('',(-0.0769897824783354,5.82191621161781E-5,-0.432610382907248));
#52690=CARTESIAN_POINT('',(-0.0769776111042551,6.21574435400559E-5,-0.437639617092753));
#52691=CARTESIAN_POINT('',(-0.076925,-9.42059550244101E-18,-0.2904));
#52692=CARTESIAN_POINT('Ctrl Pts',(-0.0769897824783354,5.82191621161781E-5,
-0.432610382907248));
#52693=CARTESIAN_POINT('Ctrl Pts',(-0.0770213613227461,0.00381177252221594,
-0.432882865044754));
#52694=CARTESIAN_POINT('Ctrl Pts',(-0.0767705832646258,0.00756108964264168,
-0.433155347182259));
#52695=CARTESIAN_POINT('Ctrl Pts',(-0.0762228831071107,0.0112665186516345,
-0.433427829319765));
#52696=CARTESIAN_POINT('Ctrl Pts',(-0.0724997739982054,0.0364549658457594,
-0.435280085000619));
#52697=CARTESIAN_POINT('Ctrl Pts',(-0.0550562160586267,0.0596153909141568,
-0.437132340681473));
#52698=CARTESIAN_POINT('Ctrl Pts',(-0.0318750171218392,0.070148739350433,
-0.438984596362327));
#52699=CARTESIAN_POINT('Ctrl Pts',(-0.00869381818505173,0.0806820877867091,
-0.44083685204318));
#52700=CARTESIAN_POINT('Ctrl Pts',(0.0202250217489445,0.078588359590864,
-0.442689107724034));
#52701=CARTESIAN_POINT('Ctrl Pts',(0.041647187712571,0.0648257210299977,
-0.444541363404887));
#52702=CARTESIAN_POINT('Ctrl Pts',(0.0630693536761977,0.0510630824691312,
-0.446393619085741));
#52703=CARTESIAN_POINT('Ctrl Pts',(0.0769948456694544,0.0256315335432433,
-0.448245874766595));
#52704=CARTESIAN_POINT('Ctrl Pts',(0.0770508509581164,0.000169477937355909,
-0.450098130447449));
#52705=CARTESIAN_POINT('Ctrl Pts',(0.0771068562467784,-0.0252925776685313,
-0.451950386128303));
#52706=CARTESIAN_POINT('Ctrl Pts',(0.0632933748308458,-0.0507851399544181,
-0.453802641809156));
#52707=CARTESIAN_POINT('Ctrl Pts',(0.0419319594279733,-0.0646418836062034,
-0.45565489749001));
#52708=CARTESIAN_POINT('Ctrl Pts',(0.0205705440251007,-0.0784986272579888,
-0.457507153170863));
#52709=CARTESIAN_POINT('Ctrl Pts',(-0.00833880536471181,-0.0807195522756726,
-0.459359408851717));
#52710=CARTESIAN_POINT('Ctrl Pts',(-0.0315661173541412,-0.0702882820528092,
-0.461211664532571));
#52711=CARTESIAN_POINT('Ctrl Pts',(-0.0547934293435706,-0.0598570118299457,
-0.463063920213425));
#52712=CARTESIAN_POINT('Ctrl Pts',(-0.0723387039326168,-0.0367735463665349,
-0.464916175894278));
#52713=CARTESIAN_POINT('Ctrl Pts',(-0.0761725832720322,-0.011601721403326,
-0.466768431575132));
#52714=CARTESIAN_POINT('Ctrl Pts',(-0.0767534857630434,-0.00778773183038919,
-0.467049082019171));
#52715=CARTESIAN_POINT('Ctrl Pts',(-0.0770196052710104,-0.00392579819187431,
-0.467329732463209));
#52716=CARTESIAN_POINT('Ctrl Pts',(-0.0769866657903101,-5.93158920058345E-5,
-0.467610382907248));
#52717=CARTESIAN_POINT('Ctrl Pts',(-0.0769983882791968,-5.48405244063995E-5,
-0.472639617092753));
#52718=CARTESIAN_POINT('Ctrl Pts',(-0.0770260911774007,-0.00348800255141457,
-0.47239032050151));
#52719=CARTESIAN_POINT('Ctrl Pts',(-0.0768163459113883,-0.00691775903718454,
-0.472141023910266));
#52720=CARTESIAN_POINT('Ctrl Pts',(-0.0763576196212321,-0.0103138848938282,
-0.471891727319023));
#52721=CARTESIAN_POINT('Ctrl Pts',(-0.0729493163922906,-0.0355468549055254,
-0.470039471638169));
#52722=CARTESIAN_POINT('Ctrl Pts',(-0.0557963076462339,-0.0589232854669328,
-0.468187215957315));
#52723=CARTESIAN_POINT('Ctrl Pts',(-0.0327484398723308,-0.0697452642775618,
-0.466334960276461));
#52724=CARTESIAN_POINT('Ctrl Pts',(-0.00970057209842773,-0.0805672430881908,
-0.464482704595607));
#52725=CARTESIAN_POINT('Ctrl Pts',(0.0192421547033216,-0.0788347701480414,
-0.462630448914754));
#52726=CARTESIAN_POINT('Ctrl Pts',(0.0408344964221166,-0.0653406912587224,
-0.460778193233901));
#52727=CARTESIAN_POINT('Ctrl Pts',(0.0624268381409117,-0.0518466123694032,
-0.458925937553047));
#52728=CARTESIAN_POINT('Ctrl Pts',(0.0766687947767522,-0.0265909275309141,
-0.457073681872193));
#52729=CARTESIAN_POINT('Ctrl Pts',(0.077042726683417,-0.00113155689853747,
-0.455221426191339));
#52730=CARTESIAN_POINT('Ctrl Pts',(0.0774166585900817,0.0243278137338391,
-0.453369170510485));
#52731=CARTESIAN_POINT('Ctrl Pts',(0.0639225657675707,0.0499908701601033,
-0.451516914829632));
#52732=CARTESIAN_POINT('Ctrl Pts',(0.0427358375238719,0.0641132616844177,
-0.449664659148778));
#52733=CARTESIAN_POINT('Ctrl Pts',(0.0215491092801732,0.0782356532087321,
-0.447812403467925));
#52734=CARTESIAN_POINT('Ctrl Pts',(-0.00733025438471345,0.0808173798310969,
-0.445960147787071));
#52735=CARTESIAN_POINT('Ctrl Pts',(-0.0306860045756403,0.0706769498119031,
-0.444107892106217));
#52736=CARTESIAN_POINT('Ctrl Pts',(-0.0540417547665674,0.0605365197927092,
-0.442255636425363));
#52737=CARTESIAN_POINT('Ctrl Pts',(-0.0718738914835347,0.0376739331319566,
-0.44040338074451));
#52738=CARTESIAN_POINT('Ctrl Pts',(-0.0760217789291502,0.0125519424202647,
-0.438551125063656));
#52739=CARTESIAN_POINT('Ctrl Pts',(-0.0767021804000287,0.00843103999565815,
-0.438247289073355));
#52740=CARTESIAN_POINT('Ctrl Pts',(-0.0770143702100962,0.00424934220686737,
-0.437943453083054));
#52741=CARTESIAN_POINT('Ctrl Pts',(-0.0769776111042551,6.21574435400559E-5,
-0.437639617092753));
#52742=CARTESIAN_POINT('Origin',(0.,0.,-0.2904));
#52743=CARTESIAN_POINT('',(-0.0768048397279485,2.24810141056936E-5,-0.397610382907248));
#52744=CARTESIAN_POINT('',(-0.0768016249961445,1.56088566556244E-5,-0.402639617092753));
#52745=CARTESIAN_POINT('',(-0.076925,-9.42059550244101E-18,-0.2904));
#52746=CARTESIAN_POINT('Ctrl Pts',(-0.0768048397279485,2.24810141056936E-5,
-0.397610382907248));
#52747=CARTESIAN_POINT('Ctrl Pts',(-0.0768348080986574,0.0114654674856241,
-0.398435997626298));
#52748=CARTESIAN_POINT('Ctrl Pts',(-0.0744407065702995,0.0228965349070991,
-0.399261612345349));
#52749=CARTESIAN_POINT('Ctrl Pts',(-0.0695589566944398,0.0331423278363428,
-0.400087227064399));
#52750=CARTESIAN_POINT('Ctrl Pts',(-0.0586068155426079,0.056128628492264,
-0.401939482745252));
#52751=CARTESIAN_POINT('Ctrl Pts',(-0.0351337611659022,0.0731491667124345,
-0.403791738426106));
#52752=CARTESIAN_POINT('Ctrl Pts',(-0.00988191866549493,0.0764147239363237,
-0.40564399410696));
#52753=CARTESIAN_POINT('Ctrl Pts',(0.0153699238349123,0.0796802811602129,
-0.407496249787814));
#52754=CARTESIAN_POINT('Ctrl Pts',(0.0424005544590212,0.0691908573878207,
-0.409348505468667));
#52755=CARTESIAN_POINT('Ctrl Pts',(0.0588397715697832,0.0497467951974147,
-0.411200761149521));
#52756=CARTESIAN_POINT('Ctrl Pts',(0.0752789886805451,0.0303027330070088,
-0.413053016830375));
#52757=CARTESIAN_POINT('Ctrl Pts',(0.0811267922779602,0.00190403239858913,
-0.414905272511229));
#52758=CARTESIAN_POINT('Ctrl Pts',(0.0737070143245067,-0.0224530263064039,
-0.416757528192082));
#52759=CARTESIAN_POINT('Ctrl Pts',(0.0662872363710531,-0.0468100850113971,
-0.418609783872936));
#52760=CARTESIAN_POINT('Ctrl Pts',(0.0455998768667307,-0.0671255018129637,
-0.420462039553789));
#52761=CARTESIAN_POINT('Ctrl Pts',(0.0211122254254216,-0.0741022016416912,
-0.422314295234643));
#52762=CARTESIAN_POINT('Ctrl Pts',(-0.00337542601588727,-0.0810789014704186,
-0.424166550915497));
#52763=CARTESIAN_POINT('Ctrl Pts',(-0.0316633693941828,-0.0747168843263072,
-0.426018806596351));
#52764=CARTESIAN_POINT('Ctrl Pts',(-0.0508060109442149,-0.0579276410943254,
-0.427871062277204));
#52765=CARTESIAN_POINT('Ctrl Pts',(-0.0671326115227027,-0.0436082344676476,
-0.429450835820552));
#52766=CARTESIAN_POINT('Ctrl Pts',(-0.0768066973653582,-0.0217038102542308,
-0.4310306093639));
#52767=CARTESIAN_POINT('Ctrl Pts',(-0.0769897824783354,5.82191621161781E-5,
-0.432610382907248));
#52768=CARTESIAN_POINT('Ctrl Pts',(-0.0769776111042551,6.21574435400559E-5,
-0.437639617092753));
#52769=CARTESIAN_POINT('Ctrl Pts',(-0.076790278052515,-0.021276721236018,
-0.4360911974022));
#52770=CARTESIAN_POINT('Ctrl Pts',(-0.0675401784708066,-0.0427581054999571,
-0.434542777711647));
#52771=CARTESIAN_POINT('Ctrl Pts',(-0.0517768802514736,-0.0570615176522107,
-0.432994358021095));
#52772=CARTESIAN_POINT('Ctrl Pts',(-0.0329204559539179,-0.074171592250363,
-0.431142102340241));
#52773=CARTESIAN_POINT('Ctrl Pts',(-0.00474396918454293,-0.0810103466840368,
-0.429289846659387));
#52774=CARTESIAN_POINT('Ctrl Pts',(0.0198579929404242,-0.0744481177684896,
-0.427437590978534));
#52775=CARTESIAN_POINT('Ctrl Pts',(0.0444599550653912,-0.0678858888529424,
-0.42558533529768));
#52776=CARTESIAN_POINT('Ctrl Pts',(0.0654873925459503,-0.0479226765881743,
-0.423733079616826));
#52777=CARTESIAN_POINT('Ctrl Pts',(0.0733173836702959,-0.0236943743820276,
-0.421880823935973));
#52778=CARTESIAN_POINT('Ctrl Pts',(0.0811473747946415,0.000533927824119099,
-0.420028568255119));
#52779=CARTESIAN_POINT('Ctrl Pts',(0.0757799195627735,0.0290273199716446,
-0.418176312574265));
#52780=CARTESIAN_POINT('Ctrl Pts',(0.0596713611069964,0.0487461874240278,
-0.416324056893412));
#52781=CARTESIAN_POINT('Ctrl Pts',(0.0435628026512191,0.0684650548764111,
-0.414471801212558));
#52782=CARTESIAN_POINT('Ctrl Pts',(0.0167131409715328,0.0794093976336524,
-0.412619545531704));
#52783=CARTESIAN_POINT('Ctrl Pts',(-0.00859024028526444,0.0765706856200469,
-0.41076728985085));
#52784=CARTESIAN_POINT('Ctrl Pts',(-0.0338936215420614,0.0737319736064415,
-0.408915034169997));
#52785=CARTESIAN_POINT('Ctrl Pts',(-0.0576507223759692,0.0571102068219895,
-0.407062778489143));
#52786=CARTESIAN_POINT('Ctrl Pts',(-0.0689894276722951,0.0343121114815454,
-0.405210522808289));
#52787=CARTESIAN_POINT('Ctrl Pts',(-0.0742354172971678,0.0237642959684653,
-0.404353554236444));
#52788=CARTESIAN_POINT('Ctrl Pts',(-0.0768231717031437,0.0118943987064725,
-0.403496585664598));
#52789=CARTESIAN_POINT('Ctrl Pts',(-0.0768016249961445,1.56088566556244E-5,
-0.402639617092753));
#52790=CARTESIAN_POINT('Origin',(0.,0.,-0.2904));
#52791=CARTESIAN_POINT('',(-0.0769074003423832,-7.00577226088184E-5,-0.362610382907248));
#52792=CARTESIAN_POINT('',(-0.0769203613463617,-7.03313400393759E-5,-0.367639617092753));
#52793=CARTESIAN_POINT('',(-0.076925,-9.42059550244101E-18,-0.2904));
#52794=CARTESIAN_POINT('Ctrl Pts',(-0.0769074003423832,-7.00577226088184E-5,
-0.362610382907248));
#52795=CARTESIAN_POINT('Ctrl Pts',(-0.0767365258441259,0.0189751470910833,
-0.363989130207843));
#52796=CARTESIAN_POINT('Ctrl Pts',(-0.0695830537667149,0.038134992706218,
-0.365367877508438));
#52797=CARTESIAN_POINT('Ctrl Pts',(-0.0567678074694182,0.0520987368937514,
-0.366746624809032));
#52798=CARTESIAN_POINT('Ctrl Pts',(-0.0395513728512194,0.0708581023599177,
-0.368598880489886));
#52799=CARTESIAN_POINT('Ctrl Pts',(-0.012116487223219,0.0802394697255212,
-0.370451136170739));
#52800=CARTESIAN_POINT('Ctrl Pts',(0.0129816459543213,0.0759495834032349,
-0.372303391851593));
#52801=CARTESIAN_POINT('Ctrl Pts',(0.0380797791318617,0.0716596970809485,
-0.374155647532447));
#52802=CARTESIAN_POINT('Ctrl Pts',(0.0608411598589422,0.0536985570707719,
-0.376007903213301));
#52803=CARTESIAN_POINT('Ctrl Pts',(0.0708493508323878,0.0302858355908709,
-0.377860158894154));
#52804=CARTESIAN_POINT('Ctrl Pts',(0.0808575418058333,0.00687311411097037,
-0.379712414575008));
#52805=CARTESIAN_POINT('Ctrl Pts',(0.0781125430256448,-0.0219911888386541,
-0.381564670255862));
#52806=CARTESIAN_POINT('Ctrl Pts',(0.0638705659683053,-0.0430977163397371,
-0.383416925936715));
#52807=CARTESIAN_POINT('Ctrl Pts',(0.0496285889109656,-0.0642042438408205,
-0.385269181617569));
#52808=CARTESIAN_POINT('Ctrl Pts',(0.0238896335764741,-0.0775529958933619,
-0.387121437298423));
#52809=CARTESIAN_POINT('Ctrl Pts',(-0.00156721608113352,-0.0770350970958021,
-0.388973692979277));
#52810=CARTESIAN_POINT('Ctrl Pts',(-0.0270240657387409,-0.0765171982982424,
-0.39082594866013));
#52811=CARTESIAN_POINT('Ctrl Pts',(-0.0521988097194646,-0.0621326486505818,
-0.392678204340984));
#52812=CARTESIAN_POINT('Ctrl Pts',(-0.0655705677463472,-0.0404643422809157,
-0.394530460021838));
#52813=CARTESIAN_POINT('Ctrl Pts',(-0.0729820685794259,-0.0284543529895058,
-0.395557100983641));
#52814=CARTESIAN_POINT('Ctrl Pts',(-0.0767675744561234,-0.0142067210167618,
-0.396583741945445));
#52815=CARTESIAN_POINT('Ctrl Pts',(-0.0768048397279485,2.24810141056936E-5,
-0.397610382907248));
#52816=CARTESIAN_POINT('Ctrl Pts',(-0.0768016249961445,1.56088566556244E-5,
-0.402639617092753));
#52817=CARTESIAN_POINT('Ctrl Pts',(-0.0767766005548495,-0.0137804704822612,
-0.401644329983744));
#52818=CARTESIAN_POINT('Ctrl Pts',(-0.0732319934678846,-0.0275885446797342,
-0.400649042874736));
#52819=CARTESIAN_POINT('Ctrl Pts',(-0.0662444625517081,-0.0393514079285166,
-0.399653755765728));
#52820=CARTESIAN_POINT('Ctrl Pts',(-0.0532404823760513,-0.0612424081016978,
-0.397801500084874));
#52821=CARTESIAN_POINT('Ctrl Pts',(-0.0283122122659939,-0.0760499845516238,
-0.395949244404021));
#52822=CARTESIAN_POINT('Ctrl Pts',(-0.00286773707221562,-0.0769976506705498,
-0.394096988723167));
#52823=CARTESIAN_POINT('Ctrl Pts',(0.0225767381215624,-0.0779453167894759,
-0.392244733042314));
#52824=CARTESIAN_POINT('Ctrl Pts',(0.0485374183990613,-0.0650330725774021,
-0.39039247736146));
#52825=CARTESIAN_POINT('Ctrl Pts',(0.0631337503916168,-0.0441700315399829,
-0.388540221680606));
#52826=CARTESIAN_POINT('Ctrl Pts',(0.0777300823841723,-0.0233069905025635,
-0.386687965999752));
#52827=CARTESIAN_POINT('Ctrl Pts',(0.0809620660917846,0.00550684736020137,
-0.384835710318898));
#52828=CARTESIAN_POINT('Ctrl Pts',(0.0713506279884725,0.0290852197925241,
-0.382983454638045));
#52829=CARTESIAN_POINT('Ctrl Pts',(0.0617391898851602,0.0526635922248472,
-0.381131198957191));
#52830=CARTESIAN_POINT('Ctrl Pts',(0.0392843299709232,0.0710064992267279,
-0.379278943276338));
#52831=CARTESIAN_POINT('Ctrl Pts',(0.0142622104544463,0.0757195580922204,
-0.377426687595484));
#52832=CARTESIAN_POINT('Ctrl Pts',(-0.0107599090620303,0.0804326169577127,
-0.37557443191463));
#52833=CARTESIAN_POINT('Ctrl Pts',(-0.0383492881807465,0.0715158276868172,
-0.373722176233776));
#52834=CARTESIAN_POINT('Ctrl Pts',(-0.055880021589883,0.0530498380002214,
-0.371869920552923));
#52835=CARTESIAN_POINT('Ctrl Pts',(-0.0692259692662876,0.0389918903719781,
-0.370459819399532));
#52836=CARTESIAN_POINT('Ctrl Pts',(-0.0767423247315113,0.0193996048245303,
-0.369049718246142));
#52837=CARTESIAN_POINT('Ctrl Pts',(-0.0769203613463617,-7.03313400393759E-5,
-0.367639617092753));
#52838=CARTESIAN_POINT('Origin',(0.,0.,-0.2904));
#52839=CARTESIAN_POINT('',(-0.0770446167695562,2.01096196933834E-5,-0.327610382907248));
#52840=CARTESIAN_POINT('',(-0.0770389450880675,2.75992272470979E-5,-0.332639617092753));
#52841=CARTESIAN_POINT('',(-0.076925,-9.42059550244101E-18,-0.2904));
#52842=CARTESIAN_POINT('Ctrl Pts',(-0.0770446167695562,2.01096196933833E-5,
-0.327610382907248));
#52843=CARTESIAN_POINT('Ctrl Pts',(-0.0770484429332084,0.00111491216618904,
-0.327690007108533));
#52844=CARTESIAN_POINT('Ctrl Pts',(-0.0770271266597134,0.00220956238892732,
-0.327769631309819));
#52845=CARTESIAN_POINT('Ctrl Pts',(-0.0769802038809804,0.00330311387201044,
-0.327849255511104));
#52846=CARTESIAN_POINT('Ctrl Pts',(-0.0758886640970139,0.0287418236379544,
-0.329701511191958));
#52847=CARTESIAN_POINT('Ctrl Pts',(-0.0609403544790954,0.0535859586125592,
-0.331553766872812));
#52848=CARTESIAN_POINT('Ctrl Pts',(-0.0389761662627314,0.0664659372481025,
-0.333406022553666));
#52849=CARTESIAN_POINT('Ctrl Pts',(-0.0170119780463675,0.0793459158836458,
-0.335258278234519));
#52850=CARTESIAN_POINT('Ctrl Pts',(0.0119680887684414,0.0802617381801278,
-0.337110533915373));
#52851=CARTESIAN_POINT('Ctrl Pts',(0.0347016995000411,0.0687942904797893,
-0.338962789596227));
#52852=CARTESIAN_POINT('Ctrl Pts',(0.0574353102316408,0.0573268427794508,
-0.34081504527708));
#52853=CARTESIAN_POINT('Ctrl Pts',(0.073922464880031,0.0334761250822914,
-0.342667300957934));
#52854=CARTESIAN_POINT('Ctrl Pts',(0.0766180406443424,0.00815709498722714,
-0.344519556638788));
#52855=CARTESIAN_POINT('Ctrl Pts',(0.0793136164086537,-0.0171619351078373,
-0.346371812319641));
#52856=CARTESIAN_POINT('Ctrl Pts',(0.0682176132888862,-0.0439492776008071,
-0.348224068000495));
#52857=CARTESIAN_POINT('Ctrl Pts',(0.0484079666791642,-0.0599460683681405,
-0.350076323681349));
#52858=CARTESIAN_POINT('Ctrl Pts',(0.0285983200694422,-0.0759428591354739,
-0.351928579362203));
#52859=CARTESIAN_POINT('Ctrl Pts',(7.50299697655082E-5,-0.081149098177171,
-0.353780835043056));
#52860=CARTESIAN_POINT('Ctrl Pts',(-0.0241086066091563,-0.0731822207791869,
-0.35563309072391));
#52861=CARTESIAN_POINT('Ctrl Pts',(-0.048292243188078,-0.0652153433812029,
-0.357485346404764));
#52862=CARTESIAN_POINT('Ctrl Pts',(-0.068136226246245,-0.044075349543538,
-0.359337602085617));
#52863=CARTESIAN_POINT('Ctrl Pts',(-0.0745592259711298,-0.0194366708413409,
-0.361189857766471));
#52864=CARTESIAN_POINT('Ctrl Pts',(-0.0762011937769633,-0.0131380691069294,
-0.36166336614673));
#52865=CARTESIAN_POINT('Ctrl Pts',(-0.0769660844151371,-0.00661082416990631,
-0.362136874526989));
#52866=CARTESIAN_POINT('Ctrl Pts',(-0.0769074003423832,-7.00577226088184E-5,
-0.362610382907248));
#52867=CARTESIAN_POINT('Ctrl Pts',(-0.0769203613463617,-7.03313400393759E-5,
-0.367639617092753));
#52868=CARTESIAN_POINT('Ctrl Pts',(-0.0769761869125781,-0.00617536884312658,
-0.367197462565289));
#52869=CARTESIAN_POINT('Ctrl Pts',(-0.0763104994214254,-0.0122683767956985,
-0.366755308037825));
#52870=CARTESIAN_POINT('Ctrl Pts',(-0.0748767850554384,-0.0181749603711571,
-0.366313153510362));
#52871=CARTESIAN_POINT('Ctrl Pts',(-0.068870727412301,-0.0429185789536437,
-0.364460897829508));
#52872=CARTESIAN_POINT('Ctrl Pts',(-0.0493865244264695,-0.0643906260163209,
-0.362608642148654));
#52873=CARTESIAN_POINT('Ctrl Pts',(-0.0253408574380519,-0.0727647103274385,
-0.360756386467801));
#52874=CARTESIAN_POINT('Ctrl Pts',(-0.00129519044963403,-0.0811387946385562,
-0.358904130786947));
#52875=CARTESIAN_POINT('Ctrl Pts',(0.0273119405413703,-0.0764149161981138,
-0.357051875106093));
#52876=CARTESIAN_POINT('Ctrl Pts',(0.0473888698769944,-0.0607548939305632,
-0.35519961942524));
#52877=CARTESIAN_POINT('Ctrl Pts',(0.0674657992126183,-0.0450948716630129,
-0.353347363744386));
#52878=CARTESIAN_POINT('Ctrl Pts',(0.0790125268928624,-0.0184987055683546,
-0.351495108063532));
#52879=CARTESIAN_POINT('Ctrl Pts',(0.0767448495391868,0.00686222951668314,
-0.349642852382678));
#52880=CARTESIAN_POINT('Ctrl Pts',(0.0744771721855112,0.032223164601721,
-0.347790596701825));
#52881=CARTESIAN_POINT('Ctrl Pts',(0.058395089797916,0.0563488686771379,
-0.345938341020971));
#52882=CARTESIAN_POINT('Ctrl Pts',(0.035858349348866,0.068198540356131,
-0.344086085340117));
#52883=CARTESIAN_POINT('Ctrl Pts',(0.0133216088998161,0.080048212035124,
-0.342233829659264));
#52884=CARTESIAN_POINT('Ctrl Pts',(-0.0156697896106886,0.0796218513176928,
-0.34038157397841));
#52885=CARTESIAN_POINT('Ctrl Pts',(-0.0378483257040854,0.0671145764057984,
-0.338529318297556));
#52886=CARTESIAN_POINT('Ctrl Pts',(-0.0600268617974825,0.0546073014939038,
-0.336677062616703));
#52887=CARTESIAN_POINT('Ctrl Pts',(-0.0753925354737718,0.0300191123875455,
-0.334824806935849));
#52888=CARTESIAN_POINT('Ctrl Pts',(-0.0769134544945309,0.00460246047782053,
-0.332972551254995));
#52889=CARTESIAN_POINT('Ctrl Pts',(-0.0770045804849021,0.00307961965225423,
-0.332861573200914));
#52890=CARTESIAN_POINT('Ctrl Pts',(-0.0770460063361865,0.00155380479662527,
-0.332750595146834));
#52891=CARTESIAN_POINT('Ctrl Pts',(-0.0770389450880675,2.75992272470979E-5,
-0.332639617092753));
#52892=CARTESIAN_POINT('Origin',(0.,0.,-0.2904));
#52893=CARTESIAN_POINT('',(-0.0768483116041091,5.73613550720782E-5,-0.292610382907248));
#52894=CARTESIAN_POINT('',(-0.0768387410148688,5.28831155507099E-5,-0.297639617092753));
#52895=CARTESIAN_POINT('',(-0.076925,-9.42059550244101E-18,-0.2904));
#52896=CARTESIAN_POINT('Ctrl Pts',(-0.0768483116041091,5.73613550720782E-5,
-0.292610382907248));
#52897=CARTESIAN_POINT('Ctrl Pts',(-0.0769089693951514,0.00881491466990413,
-0.293243139690078));
#52898=CARTESIAN_POINT('Ctrl Pts',(-0.0755273577316007,0.0175539059982861,
-0.293875896472908));
#52899=CARTESIAN_POINT('Ctrl Pts',(-0.0726202453865263,0.0257519380010413,
-0.294508653255738));
#52900=CARTESIAN_POINT('Ctrl Pts',(-0.0641103162918734,0.0497498654211309,
-0.296360908936592));
#52901=CARTESIAN_POINT('Ctrl Pts',(-0.0425284287601913,0.0691123325583359,
-0.298213164617445));
#52902=CARTESIAN_POINT('Ctrl Pts',(-0.0177512410247428,0.0749783688332192,
-0.300065420298299));
#52903=CARTESIAN_POINT('Ctrl Pts',(0.00702594671070583,0.0808444051081026,
-0.301917675979152));
#52904=CARTESIAN_POINT('Ctrl Pts',(0.0349984346499207,0.0732140105206642,
-0.303769931660006));
#52905=CARTESIAN_POINT('Ctrl Pts',(0.0533649929234512,0.0555791317050634,
-0.30562218734086));
#52906=CARTESIAN_POINT('Ctrl Pts',(0.0717315511969815,0.0379442528894627,
-0.307474443021714));
#52907=CARTESIAN_POINT('Ctrl Pts',(0.0804921798048274,0.0103048898457,-0.309326698702568));
#52908=CARTESIAN_POINT('Ctrl Pts',(0.0756376958364942,-0.0146901776488498,
-0.311178954383421));
#52909=CARTESIAN_POINT('Ctrl Pts',(0.0707832118681609,-0.0396852451433996,
-0.313031210064275));
#52910=CARTESIAN_POINT('Ctrl Pts',(0.0523136153236482,-0.0620360170887368,
-0.314883465745128));
#52911=CARTESIAN_POINT('Ctrl Pts',(0.0286812666607068,-0.0715139657238095,
-0.316735721425982));
#52912=CARTESIAN_POINT('Ctrl Pts',(0.00504891799776517,-0.0809919143588823,
-0.318587977106836));
#52913=CARTESIAN_POINT('Ctrl Pts',(-0.0237461827836053,-0.0775970396836909,
-0.32044023278769));
#52914=CARTESIAN_POINT('Ctrl Pts',(-0.0445263481992833,-0.0628829600674536,
-0.322292488468544));
#52915=CARTESIAN_POINT('Ctrl Pts',(-0.0644132222130738,-0.0488014048101396,
-0.324065119948112));
#52916=CARTESIAN_POINT('Ctrl Pts',(-0.0769594369118439,-0.0243529004262267,
-0.32583775142768));
#52917=CARTESIAN_POINT('Ctrl Pts',(-0.0770446167695562,2.01096196933833E-5,
-0.327610382907248));
#52918=CARTESIAN_POINT('Ctrl Pts',(-0.0770389450880675,2.75992272470979E-5,
-0.332639617092753));
#52919=CARTESIAN_POINT('Ctrl Pts',(-0.0769281520716595,-0.0239190056562616,
-0.33089833946598));
#52920=CARTESIAN_POINT('Ctrl Pts',(-0.064880555867624,-0.0479617984574756,
-0.329157061839207));
#52921=CARTESIAN_POINT('Ctrl Pts',(-0.0455817838885432,-0.0621221627301428,
-0.327415784212434));
#52922=CARTESIAN_POINT('Ctrl Pts',(-0.0250530298965668,-0.0771850193152902,
-0.32556352853158));
#52923=CARTESIAN_POINT('Ctrl Pts',(0.00368064245261536,-0.0810656177724936,
-0.323711272850727));
#52924=CARTESIAN_POINT('Ctrl Pts',(0.0274696575640593,-0.071988054828878,
-0.321859017169873));
#52925=CARTESIAN_POINT('Ctrl Pts',(0.0512586726755034,-0.0629104918852623,
-0.320006761489019));
#52926=CARTESIAN_POINT('Ctrl Pts',(0.0701030305492093,-0.040874767540827,
-0.318154505808165));
#52927=CARTESIAN_POINT('Ctrl Pts',(0.0753788662859333,-0.0159652322933174,
-0.316302250127312));
#52928=CARTESIAN_POINT('Ctrl Pts',(0.0806547020226573,0.00894430295419205,
-0.314449994446458));
#52929=CARTESIAN_POINT('Ctrl Pts',(0.0723620156223999,0.0367276491047761,
-0.312597738765605));
#52930=CARTESIAN_POINT('Ctrl Pts',(0.0542958425884615,0.0546701344642687,
-0.310745483084751));
#52931=CARTESIAN_POINT('Ctrl Pts',(0.036229669554523,0.0726126198237612,
-0.308893227403897));
#52932=CARTESIAN_POINT('Ctrl Pts',(0.00839000988690367,0.0807142443921621,
-0.307040971723043));
#52933=CARTESIAN_POINT('Ctrl Pts',(-0.0164826936026276,0.0752674095232067,
-0.30518871604219));
#52934=CARTESIAN_POINT('Ctrl Pts',(-0.0413553970921589,0.0698205746542512,
-0.303336460361336));
#52935=CARTESIAN_POINT('Ctrl Pts',(-0.0632611444036019,0.0508252803479395,
-0.301484204680482));
#52936=CARTESIAN_POINT('Ctrl Pts',(-0.0721750672662027,0.0269744655155819,
-0.299631948999629));
#52937=CARTESIAN_POINT('Ctrl Pts',(-0.0753710790476155,0.0184229572318016,
-0.298967838364003));
#52938=CARTESIAN_POINT('Ctrl Pts',(-0.0768969651883808,0.00924726184010815,
-0.298303727728378));
#52939=CARTESIAN_POINT('Ctrl Pts',(-0.0768387410148688,5.28831155507099E-5,
-0.297639617092753));
#52940=CARTESIAN_POINT('Origin',(0.,0.,-0.2904));
#52941=CARTESIAN_POINT('',(-0.0768380872454154,-5.25393648240572E-5,-0.257610382907248));
#52942=CARTESIAN_POINT('',(-0.0768475938414276,-5.7058424657009E-5,-0.262639617092752));
#52943=CARTESIAN_POINT('',(-0.076925,-9.42059550244101E-18,-0.2904));
#52944=CARTESIAN_POINT('Ctrl Pts',(-0.0768380872454154,-5.25393648240572E-5,
-0.257610382907248));
#52945=CARTESIAN_POINT('Ctrl Pts',(-0.0767348490166546,0.0163660347791766,
-0.258796272271623));
#52946=CARTESIAN_POINT('Ctrl Pts',(-0.0715814297759752,0.0328437608543134,
-0.259982161635997));
#52947=CARTESIAN_POINT('Ctrl Pts',(-0.061863405086039,0.0459323574614827,
-0.261168051000372));
#52948=CARTESIAN_POINT('Ctrl Pts',(-0.0466846987249234,0.0663756029684686,
-0.263020306681225));
#52949=CARTESIAN_POINT('Ctrl Pts',(-0.0203703117315888,0.078550825357997,
-0.264872562362079));
#52950=CARTESIAN_POINT('Ctrl Pts',(0.0050373334427575,0.0768861991686106,
-0.266724818042932));
#52951=CARTESIAN_POINT('Ctrl Pts',(0.0304449786171051,0.0752215729792241,
-0.268577073723786));
#52952=CARTESIAN_POINT('Ctrl Pts',(0.054945881972464,0.0597170982109209,
-0.27042932940464));
#52953=CARTESIAN_POINT('Ctrl Pts',(0.0673275372583098,0.0374681875400943,
-0.272281585085494));
#52954=CARTESIAN_POINT('Ctrl Pts',(0.0797091925441554,0.0152192768692683,
-0.274133840766348));
#52955=CARTESIAN_POINT('Ctrl Pts',(0.0799715997604887,-0.013774069704081,
-0.275986096447201));
#52956=CARTESIAN_POINT('Ctrl Pts',(0.0679946718023306,-0.0362434401968428,
-0.277838352128055));
#52957=CARTESIAN_POINT('Ctrl Pts',(0.0560177438441725,-0.0587128106896046,
-0.279690607808908));
#52958=CARTESIAN_POINT('Ctrl Pts',(0.031801480711523,-0.074658205101779,
-0.281542863489762));
#52959=CARTESIAN_POINT('Ctrl Pts',(0.00642812691598172,-0.0767824298597068,
-0.283395119170616));
#52960=CARTESIAN_POINT('Ctrl Pts',(-0.0189452268795601,-0.0789066546176347,
-0.28524737485147));
#52961=CARTESIAN_POINT('Ctrl Pts',(-0.0454756713379933,-0.0672097097213156,
-0.287099630532323));
#52962=CARTESIAN_POINT('Ctrl Pts',(-0.0610219082383983,-0.0470445434216687,
-0.288951886213177));
#52963=CARTESIAN_POINT('Ctrl Pts',(-0.0712573303588049,-0.0337680836245259,
-0.2901713851112));
#52964=CARTESIAN_POINT('Ctrl Pts',(-0.076731407113569,-0.0168208877710075,
-0.291390884009224));
#52965=CARTESIAN_POINT('Ctrl Pts',(-0.0768483116041091,5.73613550720782E-5,
-0.292610382907248));
#52966=CARTESIAN_POINT('Ctrl Pts',(-0.0768387410148688,5.28831155507099E-5,
-0.297639617092753));
#52967=CARTESIAN_POINT('Ctrl Pts',(-0.0767345734868098,-0.0163965681347663,
-0.296451472047524));
#52968=CARTESIAN_POINT('Ctrl Pts',(-0.0715599913475533,-0.0329058209298907,
-0.295263327002296));
#52969=CARTESIAN_POINT('Ctrl Pts',(-0.0618075588824273,-0.0460074753678952,
-0.294075181957067));
#52970=CARTESIAN_POINT('Ctrl Pts',(-0.0466040292222927,-0.0664322660606102,
-0.292222926276214));
#52971=CARTESIAN_POINT('Ctrl Pts',(-0.0202748714882653,-0.0785755120876367,
-0.29037067059536));
#52972=CARTESIAN_POINT('Ctrl Pts',(0.00513073223922229,-0.0768800215362977,
-0.288518414914506));
#52973=CARTESIAN_POINT('Ctrl Pts',(0.0305363359667096,-0.0751845309849588,
-0.286666159233653));
#52974=CARTESIAN_POINT('Ctrl Pts',(0.0550183856876571,-0.0596503038552547,
-0.284813903552799));
#52975=CARTESIAN_POINT('Ctrl Pts',(0.0673730032617221,-0.0373863685884066,
-0.282961647871945));
#52976=CARTESIAN_POINT('Ctrl Pts',(0.0797276208357874,-0.0151224333215578,
-0.281109392191092));
#52977=CARTESIAN_POINT('Ctrl Pts',(0.0799548062629695,0.0138712100824353,
-0.279257136510238));
#52978=CARTESIAN_POINT('Ctrl Pts',(0.0679505912125762,0.0363260137999418,
-0.277404880829384));
#52979=CARTESIAN_POINT('Ctrl Pts',(0.0559463761621832,0.0587808175174479,
-0.275552625148531));
#52980=CARTESIAN_POINT('Ctrl Pts',(0.0317107606342153,0.0746967815484678,
-0.273700369467677));
#52981=CARTESIAN_POINT('Ctrl Pts',(0.00633484550162029,0.0767901807342762,
-0.271848113786823));
#52982=CARTESIAN_POINT('Ctrl Pts',(-0.0190410696309747,0.0788835799200847,
-0.269995858105969));
#52983=CARTESIAN_POINT('Ctrl Pts',(-0.0455572843681968,0.0671544142606818,
-0.268143602425116));
#52984=CARTESIAN_POINT('Ctrl Pts',(-0.0610790125281194,0.0469703774023803,
-0.266291346744262));
#52985=CARTESIAN_POINT('Ctrl Pts',(-0.0712793960479106,0.0337060736592007,
-0.265074103527092));
#52986=CARTESIAN_POINT('Ctrl Pts',(-0.076731592629824,0.016790366214193,
-0.263856860309922));
#52987=CARTESIAN_POINT('Ctrl Pts',(-0.0768475938414276,-5.7058424657009E-5,
-0.262639617092752));
#52988=CARTESIAN_POINT('Origin',(0.,0.,-0.2904));
#52989=CARTESIAN_POINT('',(-0.0770384785824837,-2.81238608518045E-5,-0.222610382907248));
#52990=CARTESIAN_POINT('',(-0.0770442613572831,-2.06596519778444E-5,-0.227639617092753));
#52991=CARTESIAN_POINT('',(-0.076925,-9.42059550244101E-18,-0.2904));
#52992=CARTESIAN_POINT('Ctrl Pts',(-0.0770384785824837,-2.81238608518045E-5,
-0.222610382907248));
#52993=CARTESIAN_POINT('Ctrl Pts',(-0.0769260041526005,0.0238878470797757,
-0.224349404853167));
#52994=CARTESIAN_POINT('Ctrl Pts',(-0.0649137963482565,0.0479013199546961,
-0.226088426799086));
#52995=CARTESIAN_POINT('Ctrl Pts',(-0.0456572181419577,0.0620667445766768,
-0.227827448745005));
#52996=CARTESIAN_POINT('Ctrl Pts',(-0.0251467775117378,0.0771545290001813,
-0.229679704425858));
#52997=CARTESIAN_POINT('Ctrl Pts',(0.00358215996774758,0.0810700308031899,
-0.231531960106712));
#52998=CARTESIAN_POINT('Ctrl Pts',(0.0273821855504783,0.0720213736698207,
-0.233384215787566));
#52999=CARTESIAN_POINT('Ctrl Pts',(0.0511822111332089,0.0629727165364516,
-0.23523647146842));
#53000=CARTESIAN_POINT('Ctrl Pts',(0.0700533248191852,0.0409599004667053,
-0.237088727149273));
#53001=CARTESIAN_POINT('Ctrl Pts',(0.0753594172744191,0.0160567922969925,
-0.238940982830127));
#53002=CARTESIAN_POINT('Ctrl Pts',(0.0806655097296531,-0.00884631587272035,
-0.240793238510981));
#53003=CARTESIAN_POINT('Ctrl Pts',(0.0724065809541445,-0.0366397161423994,
-0.242645494191834));
#53004=CARTESIAN_POINT('Ctrl Pts',(0.0543622177318953,-0.0546041356865831,
-0.244497749872688));
#53005=CARTESIAN_POINT('Ctrl Pts',(0.0363178545096461,-0.0725685552307669,
-0.246350005553542));
#53006=CARTESIAN_POINT('Ctrl Pts',(0.00848805684065565,-0.0807039940494551,
-0.248202261234396));
#53007=CARTESIAN_POINT('Ctrl Pts',(-0.0163912456732748,-0.0752873788631742,
-0.250054516915249));
#53008=CARTESIAN_POINT('Ctrl Pts',(-0.0412705481872051,-0.0698707636768933,
-0.251906772596103));
#53009=CARTESIAN_POINT('Ctrl Pts',(-0.0631993555460757,-0.0509020944856437,
-0.253759028276956));
#53010=CARTESIAN_POINT('Ctrl Pts',(-0.0721422463610633,-0.0270621255777965,
-0.25561128395781));
#53011=CARTESIAN_POINT('Ctrl Pts',(-0.0753595350284208,-0.0184854736445279,
-0.256277650274289));
#53012=CARTESIAN_POINT('Ctrl Pts',(-0.0768960981191831,-0.00927834499463494,
-0.256944016590769));
#53013=CARTESIAN_POINT('Ctrl Pts',(-0.0768380872454154,-5.25393648240572E-5,
-0.257610382907248));
#53014=CARTESIAN_POINT('Ctrl Pts',(-0.0768475938414276,-5.7058424657009E-5,
-0.262639617092752));
#53015=CARTESIAN_POINT('Ctrl Pts',(-0.0769081094509062,-0.00884603705747186,
-0.262004604629068));
#53016=CARTESIAN_POINT('Ctrl Pts',(-0.0755163746955851,-0.0176164324632363,
-0.261369592165385));
#53017=CARTESIAN_POINT('Ctrl Pts',(-0.0725889065436049,-0.0258401387677387,
-0.260734579701701));
#53018=CARTESIAN_POINT('Ctrl Pts',(-0.0640498308165448,-0.0498277100223563,
-0.258882324020847));
#53019=CARTESIAN_POINT('Ctrl Pts',(-0.042444437779801,-0.0691639444743909,
-0.257030068339994));
#53020=CARTESIAN_POINT('Ctrl Pts',(-0.0176601426423535,-0.0749998765771247,
-0.25517781265914));
#53021=CARTESIAN_POINT('Ctrl Pts',(0.00712415249509371,-0.0808358086798583,
-0.253325556978286));
#53022=CARTESIAN_POINT('Ctrl Pts',(0.0350873497332448,-0.0731714384332915,
-0.251473301297432));
#53023=CARTESIAN_POINT('Ctrl Pts',(0.0534324709660324,-0.0555142609713604,
-0.249621045616579));
#53024=CARTESIAN_POINT('Ctrl Pts',(0.0717775921988202,-0.0378570835094291,
-0.247768789935725));
#53025=CARTESIAN_POINT('Ctrl Pts',(0.0805046374262445,-0.0102070988321336,
-0.245916534254871));
#53026=CARTESIAN_POINT('Ctrl Pts',(0.0756197927165552,0.0147820524365676,
-0.244064278574018));
#53027=CARTESIAN_POINT('Ctrl Pts',(0.0707349480068659,0.0397712037052691,
-0.242212022893164));
#53028=CARTESIAN_POINT('Ctrl Pts',(0.0522382133600625,0.0620995215653761,
-0.24035976721231));
#53029=CARTESIAN_POINT('Ctrl Pts',(0.0285943686184854,0.0715487540635222,
-0.238507511531456));
#53030=CARTESIAN_POINT('Ctrl Pts',(0.00495052387690865,0.0809979865616681,
-0.236655255850603));
#53031=CARTESIAN_POINT('Ctrl Pts',(-0.0238404309594419,0.0775681336978536,
-0.234803000169749));
#53032=CARTESIAN_POINT('Ctrl Pts',(-0.0446027057419749,0.0628288211351049,
-0.232950744488896));
#53033=CARTESIAN_POINT('Ctrl Pts',(-0.0644471738579057,0.0487410672032344,
-0.231180368690181));
#53034=CARTESIAN_POINT('Ctrl Pts',(-0.0769570964452667,0.0243216340277852,
-0.229409992891467));
#53035=CARTESIAN_POINT('Ctrl Pts',(-0.0770442613572831,-2.06596519778444E-5,
-0.227639617092753));
#53036=CARTESIAN_POINT('Origin',(0.,0.,-0.2904));
#53037=CARTESIAN_POINT('',(-0.0769213030505415,7.03209464845075E-5,-0.187610382907248));
#53038=CARTESIAN_POINT('',(-0.0769083233862821,7.01032878403822E-5,-0.192639617092753));
#53039=CARTESIAN_POINT('',(-0.076925,-9.42059550244101E-18,-0.2904));
#53040=CARTESIAN_POINT('Ctrl Pts',(-0.0769213030505415,7.03209464845076E-5,
-0.187610382907248));
#53041=CARTESIAN_POINT('Ctrl Pts',(-0.0769768969517964,0.00614402362538094,
-0.188050281753858));
#53042=CARTESIAN_POINT('Ctrl Pts',(-0.0763180708120862,0.0122058064274764,
-0.188490180600467));
#53043=CARTESIAN_POINT('Ctrl Pts',(-0.0748988104695978,0.0180839857623078,
-0.188930079447077));
#53044=CARTESIAN_POINT('Ctrl Pts',(-0.0689228160966994,0.042834882814957,
-0.190782335127931));
#53045=CARTESIAN_POINT('Ctrl Pts',(-0.0494647117111675,0.0643305841711047,
-0.192634590808785));
#53046=CARTESIAN_POINT('Ctrl Pts',(-0.0254292349826108,0.0727338735322628,
-0.194486846489638));
#53047=CARTESIAN_POINT('Ctrl Pts',(-0.00139375825405342,0.0811371628934212,
-0.196339102170492));
#53048=CARTESIAN_POINT('Ctrl Pts',(0.027219090817529,0.0764480402595892,
-0.198191357851346));
#53049=CARTESIAN_POINT('Ctrl Pts',(0.0473150297721676,0.0608124190315364,
-0.200043613532199));
#53050=CARTESIAN_POINT('Ctrl Pts',(0.0674109687268059,0.0451767978034838,
-0.201895869213053));
#53051=CARTESIAN_POINT('Ctrl Pts',(0.0789899975645006,0.0185946779812107,
-0.203748124893907));
#53052=CARTESIAN_POINT('Ctrl Pts',(0.0767531307198992,-0.00676899368468636,
-0.20560038057476));
#53053=CARTESIAN_POINT('Ctrl Pts',(0.0745162638752978,-0.0321326653505834,
-0.207452636255614));
#53054=CARTESIAN_POINT('Ctrl Pts',(0.0584635013484002,-0.0562778888601044,
-0.209304891936468));
#53055=CARTESIAN_POINT('Ctrl Pts',(0.0359411722749404,-0.0681549300220585,
-0.211157147617321));
#53056=CARTESIAN_POINT('Ctrl Pts',(0.0134188432014803,-0.0800319711840128,
-0.213009403298175));
#53057=CARTESIAN_POINT('Ctrl Pts',(-0.0155730524185423,-0.0796408299983998,
-0.214861658979029));
#53058=CARTESIAN_POINT('Ctrl Pts',(-0.0377667666111407,-0.0671605069259333,
-0.216713914659883));
#53059=CARTESIAN_POINT('Ctrl Pts',(-0.0599604808037389,-0.054680183853467,
-0.218566170340736));
#53060=CARTESIAN_POINT('Ctrl Pts',(-0.0753560135689132,-0.0301106788941475,
-0.22041842602159));
#53061=CARTESIAN_POINT('Ctrl Pts',(-0.0769078080610228,-0.00469589289248762,
-0.222270681702444));
#53062=CARTESIAN_POINT('Ctrl Pts',(-0.077002673736431,-0.00314221368325,
-0.222383915437378));
#53063=CARTESIAN_POINT('Ctrl Pts',(-0.0770458021817116,-0.00158537546457811,
-0.222497149172313));
#53064=CARTESIAN_POINT('Ctrl Pts',(-0.0770384785824837,-2.81238608518045E-5,
-0.222610382907248));
#53065=CARTESIAN_POINT('Ctrl Pts',(-0.0770442613572831,-2.06596519778444E-5,
-0.227639617092753));
#53066=CARTESIAN_POINT('Ctrl Pts',(-0.0770482927345352,-0.0011464907545882,
-0.227557737210613));
#53067=CARTESIAN_POINT('Ctrl Pts',(-0.077025751055757,-0.00227215685099022,
-0.227475857328474));
#53068=CARTESIAN_POINT('Ctrl Pts',(-0.0769761329357462,-0.00339662817961441,
-0.227393977446334));
#53069=CARTESIAN_POINT('Ctrl Pts',(-0.0758536906182689,-0.0288339926699021,
-0.225541721765481));
#53070=CARTESIAN_POINT('Ctrl Pts',(-0.0608752112545988,-0.0536599493887943,
-0.223689466084627));
#53071=CARTESIAN_POINT('Ctrl Pts',(-0.0388953928553611,-0.0665132358208449,
-0.221837210403773));
#53072=CARTESIAN_POINT('Ctrl Pts',(-0.0169155744561231,-0.0793665222528957,
-0.21998495472292));
#53073=CARTESIAN_POINT('Ctrl Pts',(0.0120655829786826,-0.0802471383981044,
-0.218132699042066));
#53074=CARTESIAN_POINT('Ctrl Pts',(0.0347852456599467,-0.0687520822165361,
-0.216280443361212));
#53075=CARTESIAN_POINT('Ctrl Pts',(0.0575049083412103,-0.057257026034968,
-0.214428187680358));
#53076=CARTESIAN_POINT('Ctrl Pts',(0.0739630762689327,-0.033386297526623,
-0.212575931999505));
#53077=CARTESIAN_POINT('Ctrl Pts',(0.0766278920219695,-0.00806401196686029,
-0.210723676318651));
#53078=CARTESIAN_POINT('Ctrl Pts',(0.0792927077750063,0.0172582735929026,
-0.208871420637797));
#53079=CARTESIAN_POINT('Ctrl Pts',(0.0681641713533576,0.0440321162040837,
-0.207019164956944));
#53080=CARTESIAN_POINT('Ctrl Pts',(0.0483351065756888,0.0600048297810181,
-0.20516690927609));
#53081=CARTESIAN_POINT('Ctrl Pts',(0.0285060417980199,0.0759775433579526,
-0.203314653595236));
#53082=CARTESIAN_POINT('Ctrl Pts',(-2.35513356690899E-5,0.0811491279006402,
-0.201462397914382));
#53083=CARTESIAN_POINT('Ctrl Pts',(-0.0241974913166144,0.0731528778566806,
-0.199610142233529));
#53084=CARTESIAN_POINT('Ctrl Pts',(-0.0483714312975601,0.0651566278127208,
-0.197757886552675));
#53085=CARTESIAN_POINT('Ctrl Pts',(-0.0681897181257618,0.0439925431821134,
-0.195905630871822));
#53086=CARTESIAN_POINT('Ctrl Pts',(-0.074582781519945,0.0193460803647884,
-0.194053375190968));
#53087=CARTESIAN_POINT('Ctrl Pts',(-0.0762093109527435,0.0130755032228149,
-0.193582122491563));
#53088=CARTESIAN_POINT('Ctrl Pts',(-0.0769668252245155,0.00657951162457119,
-0.193110869792158));
#53089=CARTESIAN_POINT('Ctrl Pts',(-0.0769083233862821,7.01032878403821E-5,
-0.192639617092753));
#53090=CARTESIAN_POINT('Origin',(0.,0.,-0.2904));
#53091=CARTESIAN_POINT('',(-0.0768014403980194,-1.51076210625975E-5,-0.152610382907248));
#53092=CARTESIAN_POINT('',(-0.0768045683068413,-2.19932982921254E-5,-0.157639617092752));
#53093=CARTESIAN_POINT('',(-0.076925,-9.42059550244101E-18,-0.2904));
#53094=CARTESIAN_POINT('Ctrl Pts',(-0.0768014403980194,-1.51076210625975E-5,
-0.152610382907248));
#53095=CARTESIAN_POINT('Ctrl Pts',(-0.0767772777264159,0.0137497882837818,
-0.153603414335402));
#53096=CARTESIAN_POINT('Ctrl Pts',(-0.0732496519640692,0.0275262395484409,
-0.154596445763557));
#53097=CARTESIAN_POINT('Ctrl Pts',(-0.0662922196675392,0.0392709047833103,
-0.155589477191711));
#53098=CARTESIAN_POINT('Ctrl Pts',(-0.0533148423861816,0.0611776866677943,
-0.157441732872564));
#53099=CARTESIAN_POINT('Ctrl Pts',(-0.0284045786794063,0.0760155357443801,
-0.159293988553418));
#53100=CARTESIAN_POINT('Ctrl Pts',(-0.00296127301607803,0.076994111547066,
-0.161146244234272));
#53101=CARTESIAN_POINT('Ctrl Pts',(0.0224820326472499,0.0779726873497518,
-0.162998499915125));
#53102=CARTESIAN_POINT('Ctrl Pts',(0.0484583802671308,0.0650919898785382,
-0.164850755595979));
#53103=CARTESIAN_POINT('Ctrl Pts',(0.0630800465304561,0.0442466957013912,
-0.166703011276833));
#53104=CARTESIAN_POINT('Ctrl Pts',(0.0777017127937813,0.0234014015242443,
-0.168555266957687));
#53105=CARTESIAN_POINT('Ctrl Pts',(0.0809686977005509,-0.00540848935883606,
-0.17040752263854));
#53106=CARTESIAN_POINT('Ctrl Pts',(0.0713859098992575,-0.0289985209741058,
-0.172259778319394));
#53107=CARTESIAN_POINT('Ctrl Pts',(0.0618031220979642,-0.0525885525893755,
-0.174112034000248));
#53108=CARTESIAN_POINT('Ctrl Pts',(0.0393705615886079,-0.0709587249368346,
-0.175964289681101));
#53109=CARTESIAN_POINT('Ctrl Pts',(0.0143541855602173,-0.0757021776946229,
-0.177816545361955));
#53110=CARTESIAN_POINT('Ctrl Pts',(-0.0106621904681737,-0.0804456304524112,
-0.179668801042809));
#53111=CARTESIAN_POINT('Ctrl Pts',(-0.0382623820155991,-0.0715623636205283,
-0.181521056723662));
#53112=CARTESIAN_POINT('Ctrl Pts',(-0.0558155356091798,-0.053117683830011,
-0.183373312404516));
#53113=CARTESIAN_POINT('Ctrl Pts',(-0.0691999277839148,-0.0390534972131984,
-0.18478566923876));
#53114=CARTESIAN_POINT('Ctrl Pts',(-0.0767428110472438,-0.0194301518413298,
-0.186198026073004));
#53115=CARTESIAN_POINT('Ctrl Pts',(-0.0769213030505415,7.03209464845076E-5,
-0.187610382907248));
#53116=CARTESIAN_POINT('Ctrl Pts',(-0.0769083233862821,7.01032878403821E-5,
-0.192639617092753));
#53117=CARTESIAN_POINT('Ctrl Pts',(-0.0767368841284859,-0.0190056756558977,
-0.191258614111304));
#53118=CARTESIAN_POINT('Ctrl Pts',(-0.0695576680328398,-0.0381966747626404,
-0.189877611129855));
#53119=CARTESIAN_POINT('Ctrl Pts',(-0.0567044741044506,-0.0521676599175141,
-0.188496608148407));
#53120=CARTESIAN_POINT('Ctrl Pts',(-0.039465263334608,-0.0709060963784499,
-0.186644352467553));
#53121=CARTESIAN_POINT('Ctrl Pts',(-0.0120190018347582,-0.0802541282962796,
-0.184792096786699));
#53122=CARTESIAN_POINT('Ctrl Pts',(0.0130739009213669,-0.0759337555994022,
-0.182939841105846));
#53123=CARTESIAN_POINT('Ctrl Pts',(0.0381668036774915,-0.0716133829025249,
-0.181087585424992));
#53124=CARTESIAN_POINT('Ctrl Pts',(0.0609063476898911,-0.0536246055909411,
-0.179235329744138));
#53125=CARTESIAN_POINT('Ctrl Pts',(0.0708860889317149,-0.0301997437191199,
-0.177383074063285));
#53126=CARTESIAN_POINT('Ctrl Pts',(0.080865830173539,-0.00677488184729807,
-0.175530818382431));
#53127=CARTESIAN_POINT('Ctrl Pts',(0.0780857686447859,0.0220860645847622,
-0.173678562701577));
#53128=CARTESIAN_POINT('Ctrl Pts',(0.0638181618136476,0.0431752747235632,
-0.171826307020723));
#53129=CARTESIAN_POINT('Ctrl Pts',(0.0495505549825093,0.0642644848623639,
-0.16997405133987));
#53130=CARTESIAN_POINT('Ctrl Pts',(0.0237954028489864,0.0775819587079064,
-0.168121795659016));
#53131=CARTESIAN_POINT('Ctrl Pts',(-0.00166079838775686,0.0770331349059874,
-0.166269539978162));
#53132=CARTESIAN_POINT('Ctrl Pts',(-0.0271169996245001,0.0764843111040684,
-0.164417284297309));
#53133=CARTESIAN_POINT('Ctrl Pts',(-0.0522742499644634,0.0620691896546879,
-0.162565028616455));
#53134=CARTESIAN_POINT('Ctrl Pts',(-0.0656196748575325,0.0403846554565688,
-0.160712772935601));
#53135=CARTESIAN_POINT('Ctrl Pts',(-0.07300032806313,0.0283920791149677,
-0.159688387654652));
#53136=CARTESIAN_POINT('Ctrl Pts',(-0.0767681988336545,0.0141760694175307,
-0.158664002373702));
#53137=CARTESIAN_POINT('Ctrl Pts',(-0.0768045683068413,-2.19932982921254E-5,
-0.157639617092752));
#53138=CARTESIAN_POINT('Origin',(0.,0.,-0.2904));
#53139=CARTESIAN_POINT('',(-0.0769767170183498,-6.24120630863603E-5,-0.117610382907248));
#53140=CARTESIAN_POINT('',(-0.0769889244048768,-5.85269688276939E-5,-0.122639617092752));
#53141=CARTESIAN_POINT('',(-0.076925,-9.42059550244101E-18,-0.2904));
#53142=CARTESIAN_POINT('Ctrl Pts',(-0.0769767170183498,-6.24120630863603E-5,
-0.117610382907248));
#53143=CARTESIAN_POINT('Ctrl Pts',(-0.0767891818127649,0.0212460239503849,
-0.119156546916947));
#53144=CARTESIAN_POINT('Ctrl Pts',(-0.0675691351190549,0.0426968904112383,
-0.120702710926645));
#53145=CARTESIAN_POINT('Ctrl Pts',(-0.0518461623588979,0.0569985772172947,
-0.122248874936344));
#53146=CARTESIAN_POINT('Ctrl Pts',(-0.0330105372685272,0.0741315465957961,
-0.124101130617198));
#53147=CARTESIAN_POINT('Ctrl Pts',(-0.00484237846485304,0.0810045253994228,
-0.125953386298051));
#53148=CARTESIAN_POINT('Ctrl Pts',(0.0197675379063687,0.0744721880741092,
-0.127805641978905));
#53149=CARTESIAN_POINT('Ctrl Pts',(0.0443774542775902,0.0679398507487956,
-0.129657897659759));
#53150=CARTESIAN_POINT('Ctrl Pts',(0.0654291282163597,0.0480021972945419,
-0.131510153340613));
#53151=CARTESIAN_POINT('Ctrl Pts',(0.0732885466351915,0.0237834245026632,
-0.133362409021466));
#53152=CARTESIAN_POINT('Ctrl Pts',(0.0811479650540234,-0.000435348289215827,
-0.13521466470232));
#53153=CARTESIAN_POINT('Ctrl Pts',(0.0758151279529177,-0.0289352404187193,
-0.137066920383174));
#53154=CARTESIAN_POINT('Ctrl Pts',(0.0597305358875067,-0.0486736626347264,
-0.138919176064027));
#53155=CARTESIAN_POINT('Ctrl Pts',(0.0436459438220958,-0.0684120848507334,
-0.140771431744881));
#53156=CARTESIAN_POINT('Ctrl Pts',(0.0168095967923794,-0.0793890371532433,
-0.142623687425735));
#53157=CARTESIAN_POINT('Ctrl Pts',(-0.00849721479305223,-0.0765810661428619,
-0.144475943106588));
#53158=CARTESIAN_POINT('Ctrl Pts',(-0.0338040263784831,-0.0737730951324806,
-0.146328198787442));
#53159=CARTESIAN_POINT('Ctrl Pts',(-0.0575813025196296,-0.0571802008092089,
-0.148180454468296));
#53160=CARTESIAN_POINT('Ctrl Pts',(-0.068947695162233,-0.0343958963013827,
-0.150032710149149));
#53161=CARTESIAN_POINT('Ctrl Pts',(-0.074220336690712,-0.0238267145105662,
-0.150891934401849));
#53162=CARTESIAN_POINT('Ctrl Pts',(-0.0768223472423177,-0.0119252366079264,
-0.151751158654548));
#53163=CARTESIAN_POINT('Ctrl Pts',(-0.0768014403980194,-1.51076210625975E-5,
-0.152610382907248));
#53164=CARTESIAN_POINT('Ctrl Pts',(-0.0768045683068413,-2.19932982921254E-5,
-0.157639617092752));
#53165=CARTESIAN_POINT('Ctrl Pts',(-0.0768339607735931,-0.0114963438937193,
-0.156811746692848));
#53166=CARTESIAN_POINT('Ctrl Pts',(-0.0744262066756044,-0.0229589728197424,
-0.155983876292944));
#53167=CARTESIAN_POINT('Ctrl Pts',(-0.0695186422021508,-0.0332268041055519,
-0.15515600589304));
#53168=CARTESIAN_POINT('Ctrl Pts',(-0.0585385852075251,-0.0561997825226952,
-0.153303750212186));
#53169=CARTESIAN_POINT('Ctrl Pts',(-0.0350448717720988,-0.0731917924101241,
-0.151451494531333));
#53170=CARTESIAN_POINT('Ctrl Pts',(-0.0097890813327328,-0.0764266708118463,
-0.149599238850479));
#53171=CARTESIAN_POINT('Ctrl Pts',(0.0154667091066325,-0.0796615492135685,
-0.147746983169625));
#53172=CARTESIAN_POINT('Ctrl Pts',(0.0424845765499378,-0.0691392961295849,
-0.145894727488772));
#53173=CARTESIAN_POINT('Ctrl Pts',(0.058900160252147,-0.0496752780278504,
-0.144042471807918));
#53174=CARTESIAN_POINT('Ctrl Pts',(0.0753157439543566,-0.0302112599261153,
-0.142190216127064));
#53175=CARTESIAN_POINT('Ctrl Pts',(0.0811290439154697,-0.00180547680662942,
-0.140337960446211));
#53176=CARTESIAN_POINT('Ctrl Pts',(0.0736796822281447,0.0225425497946054,
-0.138485704765357));
#53177=CARTESIAN_POINT('Ctrl Pts',(0.0662303205408196,0.0468905763958403,
-0.136633449084503));
#53178=CARTESIAN_POINT('Ctrl Pts',(0.0455182972050559,0.0671808464788235,
-0.13478119340365));
#53179=CARTESIAN_POINT('Ctrl Pts',(0.0210221888861179,0.0741277930278272,
-0.132928937722796));
#53180=CARTESIAN_POINT('Ctrl Pts',(-0.00347391943281973,0.0810747395768307,
-0.131076682041942));
#53181=CARTESIAN_POINT('Ctrl Pts',(-0.031754112734932,0.0746783625918553,
-0.129224426361088));
#53182=CARTESIAN_POINT('Ctrl Pts',(-0.050876343940606,0.0578658772753876,
-0.127372170680235));
#53183=CARTESIAN_POINT('Ctrl Pts',(-0.0671622496120032,0.0435471219470607,
-0.12579465281774));
#53184=CARTESIAN_POINT('Ctrl Pts',(-0.0768054414749702,0.0216730583618212,
-0.124217134955246));
#53185=CARTESIAN_POINT('Ctrl Pts',(-0.0769889244048768,-5.85269688276939E-5,
-0.122639617092752));
#53186=CARTESIAN_POINT('Origin',(0.,0.,-0.2904));
#53187=CARTESIAN_POINT('',(-0.076999203572401,5.4492118465423E-5,-0.0826103829072478));
#53188=CARTESIAN_POINT('',(-0.0769875287350775,5.90179537171767E-5,-0.0876396170927523));
#53189=CARTESIAN_POINT('',(-0.076925,-9.42059550244101E-18,-0.2904));
#53190=CARTESIAN_POINT('Ctrl Pts',(-0.076999203572401,5.4492118465423E-5,
-0.0826103829072478));
#53191=CARTESIAN_POINT('Ctrl Pts',(-0.0770265285682266,0.00345649638462249,
-0.0828574238176373));
#53192=CARTESIAN_POINT('Ctrl Pts',(-0.0768205763822429,0.00685517124978457,
-0.0831044647280268));
#53193=CARTESIAN_POINT('Ctrl Pts',(-0.0763700887674245,0.0102211183005622,
-0.0833515056384164));
#53194=CARTESIAN_POINT('Ctrl Pts',(-0.0729924366919608,0.0354582117699201,
-0.08520376131927));
#53195=CARTESIAN_POINT('Ctrl Pts',(-0.0558678488876682,0.0588554607511704,
-0.0870560170001238));
#53196=CARTESIAN_POINT('Ctrl Pts',(-0.032833146889111,0.0697054301112457,
-0.0889082726809775));
#53197=CARTESIAN_POINT('Ctrl Pts',(-0.00979844489055356,0.0805553994713211,
-0.0907605283618312));
#53198=CARTESIAN_POINT('Ctrl Pts',(0.0191463713022683,0.0788580892102209,
-0.0926127840426848));
#53199=CARTESIAN_POINT('Ctrl Pts',(0.0407550916409124,0.0653902510666844,
-0.0944650397235385));
#53200=CARTESIAN_POINT('Ctrl Pts',(0.0623638119795563,0.051922412923148,
-0.0963172954043922));
#53201=CARTESIAN_POINT('Ctrl Pts',(0.0766364364640223,0.0266840468971758,
-0.0981695510852459));
#53202=CARTESIAN_POINT('Ctrl Pts',(0.0770412958690424,0.00122514865842206,
-0.1000218067661));
#53203=CARTESIAN_POINT('Ctrl Pts',(0.0774461552740624,-0.0242337495803313,
-0.101874062446953));
#53204=CARTESIAN_POINT('Ctrl Pts',(0.0639832495996361,-0.0499131800318667,
-0.103726318127807));
#53205=CARTESIAN_POINT('Ctrl Pts',(0.0428136930638241,-0.0640612993006833,
-0.105578573808661));
#53206=CARTESIAN_POINT('Ctrl Pts',(0.0216441365280112,-0.0782094185695004,
-0.107430829489514));
#53207=CARTESIAN_POINT('Ctrl Pts',(-0.00723207086918824,-0.0808262266555986,
-0.109283085170368));
#53208=CARTESIAN_POINT('Ctrl Pts',(-0.0306001232239576,-0.0707141769196905,
-0.111135340851222));
#53209=CARTESIAN_POINT('Ctrl Pts',(-0.0539681755787259,-0.0606021271837827,
-0.112987596532076));
#53210=CARTESIAN_POINT('Ctrl Pts',(-0.0718280728910644,-0.0377612196258701,
-0.114839852212929));
#53211=CARTESIAN_POINT('Ctrl Pts',(-0.0760064758587001,-0.0126442858702262,
-0.116692107893783));
#53212=CARTESIAN_POINT('Ctrl Pts',(-0.0766969714313918,-0.00849362551214272,
-0.116998199564938));
#53213=CARTESIAN_POINT('Ctrl Pts',(-0.0770138430697374,-0.00428080981917798,
-0.117304291236093));
#53214=CARTESIAN_POINT('Ctrl Pts',(-0.0769767170183498,-6.24120630863603E-5,
-0.117610382907248));
#53215=CARTESIAN_POINT('Ctrl Pts',(-0.0769889244048768,-5.85269688276939E-5,
-0.122639617092752));
#53216=CARTESIAN_POINT('Ctrl Pts',(-0.0770208794787732,-0.00384326277764943,
-0.122364879274393));
#53217=CARTESIAN_POINT('Ctrl Pts',(-0.0767659110702742,-0.00762367706270524,
-0.122090141456033));
#53218=CARTESIAN_POINT('Ctrl Pts',(-0.0762091386433896,-0.0113591069246425,
-0.121815403637674));
#53219=CARTESIAN_POINT('Ctrl Pts',(-0.072455433031263,-0.0365430121602462,
-0.11996314795682));
#53220=CARTESIAN_POINT('Ctrl Pts',(-0.0549837526977732,-0.059682228983493,
-0.118110892275966));
#53221=CARTESIAN_POINT('Ctrl Pts',(-0.0317897751949185,-0.0701874085460173,
-0.116258636595113));
#53222=CARTESIAN_POINT('Ctrl Pts',(-0.00859579769206384,-0.0806925881085414,
-0.114406380914259));
#53223=CARTESIAN_POINT('Ctrl Pts',(0.0203204769801554,-0.078563730410343,
-0.112554125233405));
#53224=CARTESIAN_POINT('Ctrl Pts',(0.0417259075957495,-0.0647750782738639,
-0.110701869552551));
#53225=CARTESIAN_POINT('Ctrl Pts',(0.0631313382113431,-0.0509864261373853,
-0.108849613871698));
#53226=CARTESIAN_POINT('Ctrl Pts',(0.0770259247703119,-0.0255379795626259,
-0.106997358190844));
#53227=CARTESIAN_POINT('Ctrl Pts',(0.077050998400323,-7.58751863531738E-5,
-0.10514510250999));
#53228=CARTESIAN_POINT('Ctrl Pts',(0.0770760720303342,0.0253862291899199,
-0.103292846829137));
#53229=CARTESIAN_POINT('Ctrl Pts',(0.0632316327313878,0.0508619913677072,
-0.101440591148283));
#53230=CARTESIAN_POINT('Ctrl Pts',(0.0418533999014276,0.0646927743211912,
-0.0995883354674292));
#53231=CARTESIAN_POINT('Ctrl Pts',(0.0204751670714671,0.0785235572746754,
-0.0977360797865755));
#53232=CARTESIAN_POINT('Ctrl Pts',(-0.00843685928950717,0.0807093610038558,
-0.0958838241057219));
#53233=CARTESIAN_POINT('Ctrl Pts',(-0.0316514812450822,0.0702498817851143,
-0.0940315684248682));
#53234=CARTESIAN_POINT('Ctrl Pts',(-0.054866103200657,0.0597904025663729,
-0.0921793127440145));
#53235=CARTESIAN_POINT('Ctrl Pts',(-0.0723833207508324,0.03668564039971,
-0.0903270570631607));
#53236=CARTESIAN_POINT('Ctrl Pts',(-0.0761866187557145,0.0115091769813019,
-0.088474801382307));
#53237=CARTESIAN_POINT('Ctrl Pts',(-0.0767582559537188,0.00772514454795501,
-0.0881964066191221));
#53238=CARTESIAN_POINT('Ctrl Pts',(-0.0770200928405554,0.00389431194997852,
-0.0879180118559372));
#53239=CARTESIAN_POINT('Ctrl Pts',(-0.0769875287350775,5.90179537171767E-5,
-0.0876396170927523));
#53240=CARTESIAN_POINT('Origin',(0.,0.,-0.2904));
#53241=CARTESIAN_POINT('',(-0.0768084924694757,2.79143412051236E-5,-0.0476103829072477));
#53242=CARTESIAN_POINT('',(-0.0768041739443497,2.12084165925656E-5,-0.0526396170927524));
#53243=CARTESIAN_POINT('',(-0.076925,-9.42059550244101E-18,-0.2904));
#53244=CARTESIAN_POINT('Ctrl Pts',(-0.0768084924694757,2.79143412051236E-5,
-0.0476103829072477));
#53245=CARTESIAN_POINT('Ctrl Pts',(-0.0768444791363969,0.0111170264114585,
-0.0484105563991817));
#53246=CARTESIAN_POINT('Ctrl Pts',(-0.0746012189287571,0.0221922041442296,
-0.0492107298911157));
#53247=CARTESIAN_POINT('Ctrl Pts',(-0.0700063260412132,0.0321861597049033,
-0.0500109033830497));
#53248=CARTESIAN_POINT('Ctrl Pts',(-0.0593699871226408,0.0553203439137752,
-0.0518631590639034));
#53249=CARTESIAN_POINT('Ctrl Pts',(-0.0361327054769651,0.0726609283048269,
-0.0537154147447572));
#53250=CARTESIAN_POINT('Ctrl Pts',(-0.0109280621864315,0.0762721671121984,
-0.0555676704256109));
#53251=CARTESIAN_POINT('Ctrl Pts',(0.0142765811041018,0.0798834059195699,
-0.0574199261064646));
#53252=CARTESIAN_POINT('Ctrl Pts',(0.0414485860394929,0.0697652991432615,
-0.0592721817873183));
#53253=CARTESIAN_POINT('Ctrl Pts',(0.0581527122960003,0.0505482940944206,
-0.061124437468172));
#53254=CARTESIAN_POINT('Ctrl Pts',(0.0748568385525076,0.0313312890455796,
-0.0629766931490256));
#53255=CARTESIAN_POINT('Ctrl Pts',(0.0810930861301312,0.00301538572420598,
-0.0648289488298794));
#53256=CARTESIAN_POINT('Ctrl Pts',(0.0740077005522793,-0.0214410439709651,
-0.0666812045107331));
#53257=CARTESIAN_POINT('Ctrl Pts',(0.0669223149744274,-0.0458974736661366,
-0.0685334601915868));
#53258=CARTESIAN_POINT('Ctrl Pts',(0.0465152962410998,-0.0664944297351054,
-0.0703857158724405));
#53259=CARTESIAN_POINT('Ctrl Pts',(0.0221255450337808,-0.0738059853161984,
-0.0722379715532942));
#53260=CARTESIAN_POINT('Ctrl Pts',(-0.00226420617353785,-0.0811175408972913,
-0.0740902272341478));
#53261=CARTESIAN_POINT('Ctrl Pts',(-0.0306366898548477,-0.0751436959905087,
-0.0759424829150016));
#53262=CARTESIAN_POINT('Ctrl Pts',(-0.0500075735221853,-0.0586183045583848,
-0.0777947385958553));
#53263=CARTESIAN_POINT('Ctrl Pts',(-0.066794904181321,-0.0442969542778871,
-0.0793999533663195));
#53264=CARTESIAN_POINT('Ctrl Pts',(-0.076821652061467,-0.0220509457566094,
-0.0810051681367836));
#53265=CARTESIAN_POINT('Ctrl Pts',(-0.076999203572401,5.4492118465423E-5,
-0.0826103829072478));
#53266=CARTESIAN_POINT('Ctrl Pts',(-0.0769875287350775,5.90179537171767E-5,
-0.0876396170927523));
#53267=CARTESIAN_POINT('Ctrl Pts',(-0.076803432696976,-0.0216232121982777,
-0.0860657561750835));
#53268=CARTESIAN_POINT('Ctrl Pts',(-0.0672101984381137,-0.0434480298897704,
-0.0844918952574148));
#53269=CARTESIAN_POINT('Ctrl Pts',(-0.0509902119604506,-0.0577655648933422,
-0.082918034339746));
#53270=CARTESIAN_POINT('Ctrl Pts',(-0.031901128700716,-0.0746156786794249,
-0.0810657786588923));
#53271=CARTESIAN_POINT('Ctrl Pts',(-0.00363358372165781,-0.0810677415814372,
-0.0792135229780386));
#53272=CARTESIAN_POINT('Ctrl Pts',(0.0208761571269007,-0.074169052572059,
-0.0773612672971849));
#53273=CARTESIAN_POINT('Ctrl Pts',(0.04538589797546,-0.0672703635626806,
-0.0755090116163311));
#53274=CARTESIAN_POINT('Ctrl Pts',(0.0661378346935198,-0.0470209226419106,
-0.0736567559354774));
#53275=CARTESIAN_POINT('Ctrl Pts',(0.0736351382952468,-0.0226876155441985,
-0.0718045002546237));
#53276=CARTESIAN_POINT('Ctrl Pts',(0.0811324418969736,0.00164569155351299,
-0.06995224457377));
#53277=CARTESIAN_POINT('Ctrl Pts',(0.075375112382369,0.0300628648281658,
-0.0680999888929164));
#53278=CARTESIAN_POINT('Ctrl Pts',(0.0589978879383866,0.0495591770732237,
-0.0662477332120627));
#53279=CARTESIAN_POINT('Ctrl Pts',(0.0426206634944041,0.0690554893182815,
-0.064395477531209));
#53280=CARTESIAN_POINT('Ctrl Pts',(0.0156235441210435,0.0796309405337437,
-0.0625432218503553));
#53281=CARTESIAN_POINT('Ctrl Pts',(-0.00963855596190587,0.0764458058085026,
-0.0606909661695016));
#53282=CARTESIAN_POINT('Ctrl Pts',(-0.0349006560448556,0.0732606710832615,
-0.0588387104886479));
#53283=CARTESIAN_POINT('Ctrl Pts',(-0.0584277368373945,0.0563149504173167,
-0.0569864548077942));
#53284=CARTESIAN_POINT('Ctrl Pts',(-0.0694530408221216,0.0333636478502638,
-0.0551341991269405));
#53285=CARTESIAN_POINT('Ctrl Pts',(-0.0744025960277123,0.0230601914328076,
-0.0543026717822111));
#53286=CARTESIAN_POINT('Ctrl Pts',(-0.0768326014642731,0.011546398058898,
-0.0534711444374817));
#53287=CARTESIAN_POINT('Ctrl Pts',(-0.0768041739443497,2.12084165925656E-5,
-0.0526396170927524));
#53288=CARTESIAN_POINT('Origin',(0.,0.,-0.2904));
#53289=CARTESIAN_POINT('',(-0.0769167618896329,-6.73610264414135E-5,-0.0126103829072477));
#53290=CARTESIAN_POINT('',(-0.0769126606442387,-6.94072219677582E-5,-0.0176396170927523));
#53291=CARTESIAN_POINT('',(-0.076925,-9.42059550244101E-18,-0.2904));
#53292=CARTESIAN_POINT('Ctrl Pts',(-0.0769167618896329,-6.73610264414135E-5,
-0.0126103829072477));
#53293=CARTESIAN_POINT('Ctrl Pts',(-0.0767492626789875,0.0186325472370117,
-0.0139636889807262));
#53294=CARTESIAN_POINT('Ctrl Pts',(-0.0698631593360463,0.0374386870015039,
-0.0153169950542047));
#53295=CARTESIAN_POINT('Ctrl Pts',(-0.0574675930756223,0.0513152403887189,
-0.0166703011276831));
#53296=CARTESIAN_POINT('Ctrl Pts',(-0.0405019128993307,0.0703079319504091,
-0.0185225568085369));
#53297=CARTESIAN_POINT('Ctrl Pts',(-0.0132152969986564,0.080065976703565,
-0.0203748124893906));
#53298=CARTESIAN_POINT('Ctrl Pts',(0.0119351900732871,0.0761207640746733,
-0.0222270681702443));
#53299=CARTESIAN_POINT('Ctrl Pts',(0.0370856771452302,0.0721755514457817,
-0.024079323851098));
#53300=CARTESIAN_POINT('Ctrl Pts',(0.0601000353884424,0.0545270814348429,
-0.0259315795319517));
#53301=CARTESIAN_POINT('Ctrl Pts',(0.0704302024641108,0.0312534747512865,
-0.0277838352128054));
#53302=CARTESIAN_POINT('Ctrl Pts',(0.0807603695397792,0.00797986806773009,
-0.0296360908936591));
#53303=CARTESIAN_POINT('Ctrl Pts',(0.0784063454479036,-0.0209188752884439,
-0.0314883465745128));
#53304=CARTESIAN_POINT('Ctrl Pts',(0.0644537650205357,-0.0422184446065205,
-0.0333406022553665));
#53305=CARTESIAN_POINT('Ctrl Pts',(0.0505011845931677,-0.063518013924597,
-0.0351928579362202));
#53306=CARTESIAN_POINT('Ctrl Pts',(0.0249500478303073,-0.0772184092045762,
-0.0370451136170738));
#53307=CARTESIAN_POINT('Ctrl Pts',(-0.000510915286151261,-0.0770494048566988,
-0.0388973692979275));
#53308=CARTESIAN_POINT('Ctrl Pts',(-0.0259718784026102,-0.0768804005088213,
-0.0407496249787812));
#53309=CARTESIAN_POINT('Ctrl Pts',(-0.0513426678726673,-0.0628419965330865,
-0.042601880659635));
#53310=CARTESIAN_POINT('Ctrl Pts',(-0.0650103645119611,-0.0413589025318731,
-0.0444541363404887));
#53311=CARTESIAN_POINT('Ctrl Pts',(-0.0727736233030644,-0.0291564939793202,
-0.0455062185294084));
#53312=CARTESIAN_POINT('Ctrl Pts',(-0.0767611765665022,-0.0145522453587242,
-0.0465583007183281));
#53313=CARTESIAN_POINT('Ctrl Pts',(-0.0768084924694757,2.79143412051236E-5,
-0.0476103829072477));
#53314=CARTESIAN_POINT('Ctrl Pts',(-0.0768041739443497,2.12084165925656E-5,
-0.0526396170927524));
#53315=CARTESIAN_POINT('Ctrl Pts',(-0.0767692781886113,-0.0141263571706058,
-0.051618888756628));
#53316=CARTESIAN_POINT('Ctrl Pts',(-0.073029916198227,-0.0282910951160585,
-0.0505981604205037));
#53317=CARTESIAN_POINT('Ctrl Pts',(-0.0656991356399959,-0.0402553268175926,
-0.0495774320843794));
#53318=CARTESIAN_POINT('Ctrl Pts',(-0.0523963992962273,-0.0619661144502356,
-0.0477251764035257));
#53319=CARTESIAN_POINT('Ctrl Pts',(-0.0272673994317745,-0.076430805247361,
-0.045872920722672));
#53320=CARTESIAN_POINT('Ctrl Pts',(-0.00181241292307686,-0.0770297407390354,
-0.0440206650418183));
#53321=CARTESIAN_POINT('Ctrl Pts',(0.0236425735856208,-0.0776286762307097,
-0.0421684093609646));
#53322=CARTESIAN_POINT('Ctrl Pts',(0.0494235467385634,-0.0643618564169329,
-0.0403161536801109));
#53323=CARTESIAN_POINT('Ctrl Pts',(0.0637328207573074,-0.0433008299216478,
-0.0384638979992572));
#53324=CARTESIAN_POINT('Ctrl Pts',(0.0780420947760517,-0.0222398034263625,
-0.0366116423184035));
#53325=CARTESIAN_POINT('Ctrl Pts',(0.0808796696605973,0.00661542975043124,
-0.0347593866375498));
#53326=CARTESIAN_POINT('Ctrl Pts',(0.0709457789894668,0.0300599825942979,
-0.0329071309566961));
#53327=CARTESIAN_POINT('Ctrl Pts',(0.0610118883183366,0.0535045354381642,
-0.0310548752758424));
#53328=CARTESIAN_POINT('Ctrl Pts',(0.0383065320915307,0.0715384079491035,
-0.0292026195949887));
#53329=CARTESIAN_POINT('Ctrl Pts',(0.0132227623505595,0.0759080376423198,
-0.027350363914135));
#53330=CARTESIAN_POINT('Ctrl Pts',(-0.0118610073904114,0.080277667335536,
-0.0254981082332814));
#53331=CARTESIAN_POINT('Ctrl Pts',(-0.0393231906455477,0.0709830542110295,
-0.0236458525524277));
#53332=CARTESIAN_POINT('Ctrl Pts',(-0.0566003641452171,0.052278899459558,
-0.021793596871574));
#53333=CARTESIAN_POINT('Ctrl Pts',(-0.0695159729521222,0.0382965460474998,
-0.0204089369453001));
#53334=CARTESIAN_POINT('Ctrl Pts',(-0.0767398316412204,0.0190558020251586,
-0.0190242770190262));
#53335=CARTESIAN_POINT('Ctrl Pts',(-0.0769126606442387,-6.94072219677582E-5,
-0.0176396170927523));
#53336=CARTESIAN_POINT('Origin',(0.,0.,-0.648563377523455));
#53337=CARTESIAN_POINT('',(-0.0569189037447819,-4.98475974056255E-5,-0.00106337752345494));
#53338=CARTESIAN_POINT('',(-0.056925,-6.31153998696879E-15,0.));
#53339=CARTESIAN_POINT('',(-0.056925,-6.31153998696879E-15,-0.648563377523455));
#53340=CARTESIAN_POINT('',(-0.0558909241998548,-0.0108009359356534,0.));
#53341=CARTESIAN_POINT('Ctrl Pts',(-0.0569189037447819,-4.98475974056176E-5,
-0.00106337752345494));
#53342=CARTESIAN_POINT('Ctrl Pts',(-0.056951368975225,-0.00367432337077014,
-0.000708918348970012));
#53343=CARTESIAN_POINT('Ctrl Pts',(-0.0566427552153233,-0.00729340615886513,
-0.000354459174485079));
#53344=CARTESIAN_POINT('Ctrl Pts',(-0.0559769847942903,-0.010840135857283,
-1.4644860844848E-16));
#53345=CARTESIAN_POINT('Origin',(0.,0.,0.));
#53346=CARTESIAN_POINT('Origin',(0.,0.,-0.648563377523455));
#53347=CARTESIAN_POINT('',(-0.056838783670132,2.06567939264175E-5,-0.0360633775234549));
#53348=CARTESIAN_POINT('',(-0.0569158687965329,-5.13617954007034E-5,-0.0291866224765442));
#53349=CARTESIAN_POINT('',(-0.056925,-6.31153998696879E-15,-0.648563377523455));
#53350=CARTESIAN_POINT('Ctrl Pts',(-0.056838783670132,2.06567939264176E-5,
-0.0360633775234549));
#53351=CARTESIAN_POINT('Ctrl Pts',(-0.0568037695943851,-0.0107687561526893,
-0.0350112953345353));
#53352=CARTESIAN_POINT('Ctrl Pts',(-0.0486578615942883,-0.0406028067131398,
-0.032106957464762));
#53353=CARTESIAN_POINT('Ctrl Pts',(-0.000444809717068389,-0.0672805062760264,
-0.0273503639141349));
#53354=CARTESIAN_POINT('Ctrl Pts',(0.0562792121311924,-0.036865361603442,
-0.021793596871574));
#53355=CARTESIAN_POINT('Ctrl Pts',(0.0615051915174765,0.0272904121586725,
-0.0162368298290127));
#53356=CARTESIAN_POINT('Ctrl Pts',(0.0104128674487777,0.0664703597195168,
-0.0106800627864517));
#53357=CARTESIAN_POINT('Ctrl Pts',(-0.0447246776124606,0.046752464534374,
-0.00562224535126571));
#53358=CARTESIAN_POINT('Ctrl Pts',(-0.0567949532401875,0.0137882060639156,
-0.0024166835969335));
#53359=CARTESIAN_POINT('Ctrl Pts',(-0.0569189037447819,-4.98475974056176E-5,
-0.00106337752345494));
#53360=CARTESIAN_POINT('',(-0.0286389268003753,0.0491962142519396,0.));
#53361=CARTESIAN_POINT('Origin',(0.,0.,0.));
#53362=CARTESIAN_POINT('Ctrl Pts',(-0.0569158687965329,-5.13617954006995E-5,
-0.0291866224765442));
#53363=CARTESIAN_POINT('Ctrl Pts',(-0.0569590584376293,-0.00483071542741229,
-0.0287190267219646));
#53364=CARTESIAN_POINT('Ctrl Pts',(-0.0542212221178314,-0.0284938299898704,
-0.0263991752865313));
#53365=CARTESIAN_POINT('Ctrl Pts',(-0.0212425420460525,-0.0638395728638739,
-0.0222270681702444));
#53366=CARTESIAN_POINT('Ctrl Pts',(0.0420792312090032,-0.0524733655289061,
-0.0166703011276832));
#53367=CARTESIAN_POINT('Ctrl Pts',(0.0669727390520183,0.00689708027414815,
-0.0111135340851222));
#53368=CARTESIAN_POINT('Ctrl Pts',(0.0303982238704425,0.0600019556186538,
-0.00555676704256101));
#53369=CARTESIAN_POINT('Ctrl Pts',(-0.012280390439628,0.0587191202828289,
-0.00185225568085369));
#53370=CARTESIAN_POINT('Ctrl Pts',(-0.0286389268003753,0.0491962142519396,
0.));
#53371=CARTESIAN_POINT('Origin',(0.,0.,-0.648563377523455));
#53372=CARTESIAN_POINT('',(-0.0569799111258879,4.03245218502727E-5,-0.0710633775234549));
#53373=CARTESIAN_POINT('',(-0.056835587933469,1.56943661208178E-5,-0.0641866224765442));
#53374=CARTESIAN_POINT('',(-0.056925,-6.31153998696879E-15,-0.648563377523455));
#53375=CARTESIAN_POINT('Ctrl Pts',(-0.0569799111258879,4.03245218502722E-5,
-0.0710633775234549));
#53376=CARTESIAN_POINT('Ctrl Pts',(-0.0568485218537396,-0.0163178431874584,
-0.0694581627529908));
#53377=CARTESIAN_POINT('Ctrl Pts',(-0.0408668960010946,-0.0517757393220317,
-0.0660006923016731));
#53378=CARTESIAN_POINT('Ctrl Pts',(0.0193202950553148,-0.0644481915748698,
-0.0606909661695014));
#53379=CARTESIAN_POINT('Ctrl Pts',(0.0646242745702175,-0.0187225474711557,
-0.0551341991269405));
#53380=CARTESIAN_POINT('Ctrl Pts',(0.0507796833441037,0.0441393100486048,
-0.0495774320843793));
#53381=CARTESIAN_POINT('Ctrl Pts',(-0.00954269745331579,0.0666017043901573,
-0.0440206650418183));
#53382=CARTESIAN_POINT('Ctrl Pts',(-0.0513627268784663,0.0353939340261016,
-0.0395159801881768));
#53383=CARTESIAN_POINT('Ctrl Pts',(-0.0568654140375617,0.00822667180334124,
-0.036863551015389));
#53384=CARTESIAN_POINT('Ctrl Pts',(-0.056838783670132,2.06567939264176E-5,
-0.0360633775234549));
#53385=CARTESIAN_POINT('Ctrl Pts',(-0.056835587933469,1.56943661208178E-5,
-0.0641866224765442));
#53386=CARTESIAN_POINT('Ctrl Pts',(-0.0568097648474042,-0.0104535961252809,
-0.0631658941404201));
#53387=CARTESIAN_POINT('Ctrl Pts',(-0.0490212243523883,-0.0399566598492793,
-0.0602929101234423));
#53388=CARTESIAN_POINT('Ctrl Pts',(-0.00158242957906591,-0.0672632578788742,
-0.055567670425611));
#53389=CARTESIAN_POINT('Ctrl Pts',(0.0556518335368746,-0.0378106591957688,
-0.0500109033830497));
#53390=CARTESIAN_POINT('Ctrl Pts',(0.0619513051118907,0.0262485211196931,
-0.0444541363404888));
#53391=CARTESIAN_POINT('Ctrl Pts',(0.0115449715450025,0.0662840697456999,
-0.0388973692979276));
#53392=CARTESIAN_POINT('Ctrl Pts',(-0.0442913408145573,0.0473861941886207,
-0.0338081980099462));
#53393=CARTESIAN_POINT('Ctrl Pts',(-0.0567879742109411,0.0141014173582273,
-0.0305712824028183));
#53394=CARTESIAN_POINT('Ctrl Pts',(-0.0569158687965329,-5.13617954006995E-5,
-0.0291866224765442));
#53395=CARTESIAN_POINT('Origin',(0.,0.,-0.648563377523455));
#53396=CARTESIAN_POINT('',(-0.056963270929731,-4.61853323570465E-5,-0.106063377523455));
#53397=CARTESIAN_POINT('',(-0.0569712716703839,4.36736693513254E-5,-0.0991866224765444));
#53398=CARTESIAN_POINT('',(-0.056925,-6.31153998696879E-15,-0.648563377523455));
#53399=CARTESIAN_POINT('Ctrl Pts',(-0.056963270929731,-4.61853323570488E-5,
-0.106063377523455));
#53400=CARTESIAN_POINT('Ctrl Pts',(-0.0569907444490709,-0.00316782709076371,
-0.1057572858523));
#53401=CARTESIAN_POINT('Ctrl Pts',(-0.0553373033443182,-0.0251503644672759,
-0.103598938500292));
#53402=CARTESIAN_POINT('Ctrl Pts',(-0.0267203606150653,-0.061748388075023,
-0.0995883354674292));
#53403=CARTESIAN_POINT('Ctrl Pts',(0.0373853828786833,-0.055939023097401,
-0.0940315684248681));
#53404=CARTESIAN_POINT('Ctrl Pts',(0.0672732959960052,0.00106981324138322,
-0.088474801382307));
#53405=CARTESIAN_POINT('Ctrl Pts',(0.035587791331269,0.0570994779548752,
-0.0829180343397459));
#53406=CARTESIAN_POINT('Ctrl Pts',(-0.0286702650266008,0.0608675398312384,
-0.0773612672971849));
#53407=CARTESIAN_POINT('Ctrl Pts',(-0.0557050211889429,0.0239300714199293,
-0.0734097150250878));
#53408=CARTESIAN_POINT('Ctrl Pts',(-0.0570001318004071,0.00255782979128222,
-0.0713104184338445));
#53409=CARTESIAN_POINT('Ctrl Pts',(-0.0569799111258879,4.03245218502722E-5,
-0.0710633775234549));
#53410=CARTESIAN_POINT('Ctrl Pts',(-0.0569712716703839,4.36736693513245E-5,
-0.0991866224765444));
#53411=CARTESIAN_POINT('Ctrl Pts',(-0.0568350394055926,-0.016001317574096,
-0.0976127615588758));
#53412=CARTESIAN_POINT('Ctrl Pts',(-0.0413812008133835,-0.0511591382639303,
-0.0941866449603535));
#53413=CARTESIAN_POINT('Ctrl Pts',(0.0182292914472235,-0.0647652241822597,
-0.0889082726809775));
#53414=CARTESIAN_POINT('Ctrl Pts',(0.0642989956139634,-0.0198110704839244,
-0.0833515056384163));
#53415=CARTESIAN_POINT('Ctrl Pts',(0.0515176118264206,0.0432756083068328,
-0.0777947385958553));
#53416=CARTESIAN_POINT('Ctrl Pts',(-0.00841651961310768,0.0667533162213003,
-0.0722379715532942));
#53417=CARTESIAN_POINT('Ctrl Pts',(-0.0510528083444251,0.0360439117930788,
-0.0677019328468572));
#53418=CARTESIAN_POINT('Ctrl Pts',(-0.0568566244829879,0.00854440961328914,
-0.0650181498212739));
#53419=CARTESIAN_POINT('Ctrl Pts',(-0.056835587933469,1.56943661208178E-5,
-0.0641866224765442));
#53420=CARTESIAN_POINT('Origin',(0.,0.,-0.648563377523455));
#53421=CARTESIAN_POINT('',(-0.056833565091417,-1.11797377874599E-5,-0.141063377523455));
#53422=CARTESIAN_POINT('',(-0.0569723044751072,-4.33103373571816E-5,-0.134186622476544));
#53423=CARTESIAN_POINT('',(-0.056925,-6.31153998696879E-15,-0.648563377523455));
#53424=CARTESIAN_POINT('Ctrl Pts',(-0.056833565091417,-1.11797377874701E-5,
-0.141063377523455));
#53425=CARTESIAN_POINT('Ctrl Pts',(-0.0568490362920882,-0.00882475260196868,
-0.140204153270756));
#53426=CARTESIAN_POINT('Ctrl Pts',(-0.0507726628702476,-0.0366178082310402,
-0.137492673337203));
#53427=CARTESIAN_POINT('Ctrl Pts',(-0.00741986034787437,-0.0668714195615047,
-0.132928937722796));
#53428=CARTESIAN_POINT('Ctrl Pts',(0.0521573533537793,-0.0425023714047127,
-0.127372170680235));
#53429=CARTESIAN_POINT('Ctrl Pts',(0.0639963557059561,0.0207679448567898,
-0.121815403637674));
#53430=CARTESIAN_POINT('Ctrl Pts',(0.0172612290645072,0.0650299242997547,
-0.116258636595113));
#53431=CARTESIAN_POINT('Ctrl Pts',(-0.0418279869431582,0.0506122645593998,
-0.111007961223706));
#53432=CARTESIAN_POINT('Ctrl Pts',(-0.0568244936586512,0.0157221958189843,
-0.107609541533154));
#53433=CARTESIAN_POINT('Ctrl Pts',(-0.056963270929731,-4.61853323570488E-5,
-0.106063377523455));
#53434=CARTESIAN_POINT('Ctrl Pts',(-0.0569723044751072,-4.33103373571769E-5,
-0.134186622476544));
#53435=CARTESIAN_POINT('Ctrl Pts',(-0.0569959514374928,-0.00284403943605085,
-0.133911884658185));
#53436=CARTESIAN_POINT('Ctrl Pts',(-0.0555352225271942,-0.024502253767729,
-0.131784891158972));
#53437=CARTESIAN_POINT('Ctrl Pts',(-0.0277591773719423,-0.0612884082229279,
-0.127805641978905));
#53438=CARTESIAN_POINT('Ctrl Pts',(0.0364355162536436,-0.0565623026212381,
-0.122248874936344));
#53439=CARTESIAN_POINT('Ctrl Pts',(0.0672817693522171,-6.62549929698068E-5,
-0.116692107893783));
#53440=CARTESIAN_POINT('Ctrl Pts',(0.0365468441487368,0.0564904338066607,
-0.111135340851222));
#53441=CARTESIAN_POINT('Ctrl Pts',(-0.0276384181430455,0.0613429607075467,
-0.105578573808661));
#53442=CARTESIAN_POINT('Ctrl Pts',(-0.0555124500581288,0.0245778251385385,
-0.101595667683768));
#53443=CARTESIAN_POINT('Ctrl Pts',(-0.0569953693200993,0.00288181615537408,
-0.0994650172397295));
#53444=CARTESIAN_POINT('Ctrl Pts',(-0.0569712716703839,4.36736693513245E-5,
-0.0991866224765444));
#53445=CARTESIAN_POINT('Origin',(0.,0.,-0.648563377523455));
#53446=CARTESIAN_POINT('',(-0.0569222642333711,5.20379574683919E-5,-0.176063377523455));
#53447=CARTESIAN_POINT('',(-0.0568358797642761,-1.62751836963598E-5,-0.169186622476544));
#53448=CARTESIAN_POINT('',(-0.056925,-6.31153998696879E-15,-0.648563377523455));
#53449=CARTESIAN_POINT('Ctrl Pts',(-0.0569222642333711,5.20379574683923E-5,
-0.176063377523455));
#53450=CARTESIAN_POINT('Ctrl Pts',(-0.0567901789907606,-0.0143784386554175,
-0.174651020689211));
#53451=CARTESIAN_POINT('Ctrl Pts',(-0.0438880872324678,-0.0479441447327426,
-0.171386408174114));
#53452=CARTESIAN_POINT('Ctrl Pts',(0.0125342308929026,-0.066103964613694,
-0.166269539978162));
#53453=CARTESIAN_POINT('Ctrl Pts',(0.0623349526476669,-0.0253218237929275,
-0.160712772935602));
#53454=CARTESIAN_POINT('Ctrl Pts',(0.0550821824500234,0.0386366957463386,
-0.15515600589304));
#53455=CARTESIAN_POINT('Ctrl Pts',(-0.00258581579222903,0.0672320952997525,
-0.149599238850479));
#53456=CARTESIAN_POINT('Ctrl Pts',(-0.0493360368562338,0.0393852313480028,
-0.144901696060617));
#53457=CARTESIAN_POINT('Ctrl Pts',(-0.0568156845573776,0.0101749327013848,
-0.142056408951609));
#53458=CARTESIAN_POINT('Ctrl Pts',(-0.056833565091417,-1.11797377874701E-5,
-0.141063377523455));
#53459=CARTESIAN_POINT('Ctrl Pts',(-0.0568358797642761,-1.62751836963529E-5,
-0.169186622476544));
#53460=CARTESIAN_POINT('Ctrl Pts',(-0.0568576303807177,-0.00850736920572494,
-0.168358752076641));
#53461=CARTESIAN_POINT('Ctrl Pts',(-0.0510894273931871,-0.035968134601679,
-0.165678625995883));
#53462=CARTESIAN_POINT('Ctrl Pts',(-0.00854793224978894,-0.0667365998802494,
-0.161146244234271));
#53463=CARTESIAN_POINT('Ctrl Pts',(0.0514322603095934,-0.0433769928549986,
-0.155589477191711));
#53464=CARTESIAN_POINT('Ctrl Pts',(0.0643378995797782,0.019684399569185,
-0.150032710149149));
#53465=CARTESIAN_POINT('Ctrl Pts',(0.0183568039000239,0.0647291948037812,
-0.144475943106589));
#53466=CARTESIAN_POINT('Ctrl Pts',(-0.0413216787244819,0.0512311939704846,
-0.139193913882386));
#53467=CARTESIAN_POINT('Ctrl Pts',(-0.0568365259143696,0.0160382040590988,
-0.135764140339039));
#53468=CARTESIAN_POINT('Ctrl Pts',(-0.0569723044751072,-4.33103373571769E-5,
-0.134186622476544));
#53469=CARTESIAN_POINT('Origin',(0.,0.,-0.648563377523455));
#53470=CARTESIAN_POINT('',(-0.0570089748886303,-2.08118398348977E-5,-0.211063377523455));
#53471=CARTESIAN_POINT('',(-0.0569126591974534,5.18768886537315E-5,-0.204186622476544));
#53472=CARTESIAN_POINT('',(-0.056925,-6.31153998696879E-15,-0.648563377523455));
#53473=CARTESIAN_POINT('Ctrl Pts',(-0.0570089748886303,-2.08118398349025E-5,
-0.211063377523455));
#53474=CARTESIAN_POINT('Ctrl Pts',(-0.057014394399661,-0.00117318814847394,
-0.210950143788521));
#53475=CARTESIAN_POINT('Ctrl Pts',(-0.0564604142361575,-0.0211706048259219,
-0.208984654372732));
#53476=CARTESIAN_POINT('Ctrl Pts',(-0.0329783512134566,-0.0586452848315629,
-0.20516690927609));
#53477=CARTESIAN_POINT('Ctrl Pts',(0.0313842223908242,-0.059513625890684,
-0.199610142233529));
#53478=CARTESIAN_POINT('Ctrl Pts',(0.0670216682215793,-0.00591075887945832,
-0.194053375190967));
#53479=CARTESIAN_POINT('Ctrl Pts',(0.0413159984164774,0.0531020654643655,
-0.188496608148407));
#53480=CARTESIAN_POINT('Ctrl Pts',(-0.0222050844590437,0.0635120091470762,
-0.182939841105846));
#53481=CARTESIAN_POINT('Ctrl Pts',(-0.0544230314477119,0.0279202910097429,
-0.178795430897528));
#53482=CARTESIAN_POINT('Ctrl Pts',(-0.0569634040816515,0.00454661741793302,
-0.176503276370065));
#53483=CARTESIAN_POINT('Ctrl Pts',(-0.0569222642333711,5.20379574683923E-5,
-0.176063377523455));
#53484=CARTESIAN_POINT('Ctrl Pts',(-0.0569126591974534,5.18768886537324E-5,
-0.204186622476544));
#53485=CARTESIAN_POINT('Ctrl Pts',(-0.0567857930323549,-0.0140643235191736,
-0.202805619495096));
#53486=CARTESIAN_POINT('Ctrl Pts',(-0.0443475684573707,-0.0473133514809718,
-0.199572360832794));
#53487=CARTESIAN_POINT('Ctrl Pts',(0.0114162724268508,-0.0663061809579219,
-0.194486846489638));
#53488=CARTESIAN_POINT('Ctrl Pts',(0.0618985035444009,-0.0263707445538147,
-0.188930079447077));
#53489=CARTESIAN_POINT('Ctrl Pts',(0.0557267127407225,0.0377011192997421,
-0.183373312404516));
#53490=CARTESIAN_POINT('Ctrl Pts',(-0.00145022720861101,0.067266170921093,
-0.177816545361955));
#53491=CARTESIAN_POINT('Ctrl Pts',(-0.048979108510772,0.040032089808678,
-0.173087648719298));
#53492=CARTESIAN_POINT('Ctrl Pts',(-0.0568089661177235,0.0104903835111149,
-0.170211007757494));
#53493=CARTESIAN_POINT('Ctrl Pts',(-0.0568358797642761,-1.62751836963529E-5,
-0.169186622476544));
#53494=CARTESIAN_POINT('Origin',(0.,0.,-0.648563377523455));
#53495=CARTESIAN_POINT('',(-0.0568606839966886,-3.88794714720325E-5,-0.246063377523455));
#53496=CARTESIAN_POINT('',(-0.057013254179569,-1.52882767560647E-5,-0.239186622476545));
#53497=CARTESIAN_POINT('',(-0.056925,-6.31153998696879E-15,-0.648563377523455));
#53498=CARTESIAN_POINT('Ctrl Pts',(-0.0568606839966886,-3.8879471472038E-5,
-0.246063377523455));
#53499=CARTESIAN_POINT('Ctrl Pts',(-0.0569036124203374,-0.00686603560376843,
-0.245397011206976));
#53500=CARTESIAN_POINT('Ctrl Pts',(-0.0526059144902416,-0.0326179607792761,
-0.242878389209643));
#53501=CARTESIAN_POINT('Ctrl Pts',(-0.0143130139311376,-0.0657417577643039,
-0.238507511531456));
#53502=CARTESIAN_POINT('Ctrl Pts',(0.0474696795615072,-0.0476809249497236,
-0.232950744488896));
#53503=CARTESIAN_POINT('Ctrl Pts',(0.0658046624882197,0.0140209656067212,
-0.227393977446334));
#53504=CARTESIAN_POINT('Ctrl Pts',(0.0239104221278329,0.0628898465207396,
-0.221837210403774));
#53505=CARTESIAN_POINT('Ctrl Pts',(-0.0385687185501853,0.0543744885075883,
-0.216393677096147));
#53506=CARTESIAN_POINT('Ctrl Pts',(-0.0569257430794525,0.0176771621061551,
-0.212802399469374));
#53507=CARTESIAN_POINT('Ctrl Pts',(-0.0570089748886303,-2.08118398349025E-5,
-0.211063377523455));
#53508=CARTESIAN_POINT('Ctrl Pts',(-0.0570132541795689,-1.52882767560661E-5,
-0.239186622476545));
#53509=CARTESIAN_POINT('Ctrl Pts',(-0.0570162374249387,-0.000848410610404804,
-0.239104742594405));
#53510=CARTESIAN_POINT('Ctrl Pts',(-0.0566222054253004,-0.020525226487873,
-0.237170607031412));
#53511=CARTESIAN_POINT('Ctrl Pts',(-0.0339638799205846,-0.0580800806653254,
-0.233384215787566));
#53512=CARTESIAN_POINT('Ctrl Pts',(0.0303748547031255,-0.0600350656792724,
-0.227827448745005));
#53513=CARTESIAN_POINT('Ctrl Pts',(0.066912308428919,-0.00704158292317649,
-0.222270681702444));
#53514=CARTESIAN_POINT('Ctrl Pts',(0.0422067405718221,0.0523968697505238,
-0.216713914659883));
#53515=CARTESIAN_POINT('Ctrl Pts',(-0.0211295124981265,0.0638778882786663,
-0.211157147617322));
#53516=CARTESIAN_POINT('Ctrl Pts',(-0.0541920864480305,0.0285701384591516,
-0.206981383556209));
#53517=CARTESIAN_POINT('Ctrl Pts',(-0.0569559509379992,0.00486888136793312,
-0.20465787517595));
#53518=CARTESIAN_POINT('Ctrl Pts',(-0.0569126591974534,5.18768886537324E-5,
-0.204186622476544));
#53519=CARTESIAN_POINT('Origin',(0.,0.,-0.648563377523455));
#53520=CARTESIAN_POINT('',(-0.0568682500885786,4.24477755887524E-5,-0.281063377523455));
#53521=CARTESIAN_POINT('',(-0.056867718939529,-4.22236051248123E-5,-0.274186622476545));
#53522=CARTESIAN_POINT('',(-0.056925,-6.31153998696879E-15,-0.648563377523455));
#53523=CARTESIAN_POINT('Ctrl Pts',(-0.0568682500885786,4.24477755887522E-5,
-0.281063377523455));
#53524=CARTESIAN_POINT('Ctrl Pts',(-0.0567817400057179,-0.012447566283586,
-0.279843878625431));
#53525=CARTESIAN_POINT('Ctrl Pts',(-0.0465781847879718,-0.0440367559175842,
-0.276772124046554));
#53526=CARTESIAN_POINT('Ctrl Pts',(0.0056131103110498,-0.0670472525489997,
-0.271848113786823));
#53527=CARTESIAN_POINT('Ctrl Pts',(0.0593736866708568,-0.0316481660265529,
-0.266291346744262));
#53528=CARTESIAN_POINT('Ctrl Pts',(0.0587911375337822,0.0327176287224069,
-0.2607345797017));
#53529=CARTESIAN_POINT('Ctrl Pts',(0.00439865432921479,0.0671378650377374,
-0.25517781265914));
#53530=CARTESIAN_POINT('Ctrl Pts',(-0.0470142696024862,0.0433499735423753,
-0.250287411933058));
#53531=CARTESIAN_POINT('Ctrl Pts',(-0.0567842870363749,0.0121109721131533,
-0.24724926688783));
#53532=CARTESIAN_POINT('Ctrl Pts',(-0.0568606839966886,-3.8879471472038E-5,
-0.246063377523455));
#53533=CARTESIAN_POINT('Ctrl Pts',(-0.056867718939529,-4.22236051248167E-5,
-0.274186622476545));
#53534=CARTESIAN_POINT('Ctrl Pts',(-0.0569125008838839,-0.00654612492033858,
-0.273551610012861));
#53535=CARTESIAN_POINT('Ctrl Pts',(-0.0528785336578182,-0.031967267484468,
-0.271064341868323));
#53536=CARTESIAN_POINT('Ctrl Pts',(-0.0154210285602653,-0.0654907076423372,
-0.266724818042933));
#53537=CARTESIAN_POINT('Ctrl Pts',(0.0466578145771441,-0.0484756562434736,
-0.261168051000371));
#53538=CARTESIAN_POINT('Ctrl Pts',(0.0660320251551521,0.0129078489013458,
-0.255611283957811));
#53539=CARTESIAN_POINT('Ctrl Pts',(0.024968913561939,0.062477149942095,
-0.250054516915249));
#53540=CARTESIAN_POINT('Ctrl Pts',(-0.0380057476550708,0.0549750082677155,
-0.244579629754827));
#53541=CARTESIAN_POINT('Ctrl Pts',(-0.0569487515781217,0.0179981672672241,
-0.240956998275259));
#53542=CARTESIAN_POINT('Ctrl Pts',(-0.0570132541795689,-1.52882767560661E-5,
-0.239186622476545));
#53543=CARTESIAN_POINT('Origin',(0.,0.,-0.648563377523455));
#53544=CARTESIAN_POINT('',(-0.0570135171869611,1.48812492774907E-5,-0.316063377523455));
#53545=CARTESIAN_POINT('',(-0.0568611677903335,3.91338492306513E-5,-0.309186622476545));
#53546=CARTESIAN_POINT('',(-0.056925,-6.31153998696879E-15,-0.648563377523455));
#53547=CARTESIAN_POINT('Ctrl Pts',(-0.0570135171869611,1.48812492774924E-5,
-0.316063377523455));
#53548=CARTESIAN_POINT('Ctrl Pts',(-0.0569504835385972,-0.018021304605307,
-0.314290746043887));
#53549=CARTESIAN_POINT('Ctrl Pts',(-0.0379648854061764,-0.0550180793549962,
-0.310665858883465));
#53550=CARTESIAN_POINT('Ctrl Pts',(0.0250447938771848,-0.0624467723856301,
-0.30518871604219));
#53551=CARTESIAN_POINT('Ctrl Pts',(0.0660476583541301,-0.0128276228378236,
-0.299631948999629));
#53552=CARTESIAN_POINT('Ctrl Pts',(0.0465988920167232,0.0485323020734347,
-0.294075181957067));
#53553=CARTESIAN_POINT('Ctrl Pts',(-0.0155005766582128,0.0654719268465212,
-0.288518414914507));
#53554=CARTESIAN_POINT('Ctrl Pts',(-0.0528978808086814,0.0319204558933633,
-0.284181146769969));
#53555=CARTESIAN_POINT('Ctrl Pts',(-0.0569131372482161,0.00652309415123876,
-0.281696134306285));
#53556=CARTESIAN_POINT('Ctrl Pts',(-0.0568682500885786,4.24477755887522E-5,
-0.281063377523455));
#53557=CARTESIAN_POINT('Ctrl Pts',(-0.0568611677903335,3.91338492306548E-5,
-0.309186622476545));
#53558=CARTESIAN_POINT('Ctrl Pts',(-0.0567840831424961,-0.0121335669947618,
-0.307998477431316));
#53559=CARTESIAN_POINT('Ctrl Pts',(-0.0469852991097598,-0.043396111163104,
-0.304958076705234));
#53560=CARTESIAN_POINT('Ctrl Pts',(0.00448021117374274,-0.0671324706620369,
-0.300065420298299));
#53561=CARTESIAN_POINT('Ctrl Pts',(0.0588308389422806,-0.0326461835242353,
-0.294508653255737));
#53562=CARTESIAN_POINT('Ctrl Pts',(0.0593351950206278,0.0317202701945406,
-0.288951886213177));
#53563=CARTESIAN_POINT('Ctrl Pts',(0.00553165596584969,0.067054020696943,
-0.283395119170615));
#53564=CARTESIAN_POINT('Ctrl Pts',(-0.0466077501799208,0.04399070875264,
-0.278473364591738));
#53565=CARTESIAN_POINT('Ctrl Pts',(-0.056781877288955,0.0124249801331489,
-0.275403865693715));
#53566=CARTESIAN_POINT('Ctrl Pts',(-0.056867718939529,-4.22236051248167E-5,
-0.274186622476545));
#53567=CARTESIAN_POINT('Origin',(0.,0.,-0.648563377523455));
#53568=CARTESIAN_POINT('',(-0.0569119761389687,-5.18431700991948E-5,-0.351063377523455));
#53569=CARTESIAN_POINT('',(-0.0570093201057945,2.04236075452674E-5,-0.344186622476545));
#53570=CARTESIAN_POINT('',(-0.056925,-6.31153998696879E-15,-0.648563377523455));
#53571=CARTESIAN_POINT('Ctrl Pts',(-0.0569119761389687,-5.18431700991979E-5,
-0.351063377523455));
#53572=CARTESIAN_POINT('Ctrl Pts',(-0.0569554027342431,-0.00489205285501732,
-0.350589869143196));
#53573=CARTESIAN_POINT('Ctrl Pts',(-0.0541752230501154,-0.0286169003842717,
-0.348264105082084));
#53574=CARTESIAN_POINT('Ctrl Pts',(-0.0210518974052001,-0.0639035108376226,
-0.344086085340117));
#53575=CARTESIAN_POINT('Ctrl Pts',(0.0422703628063335,-0.0523455586459296,
-0.338529318297556));
#53576=CARTESIAN_POINT('Ctrl Pts',(0.0669037060988672,0.00712286402858384,
-0.332972551254995));
#53577=CARTESIAN_POINT('Ctrl Pts',(0.0303019012879613,0.0600719223936441,
-0.327415784212435));
#53578=CARTESIAN_POINT('Ctrl Pts',(-0.0340344121380907,0.0580387790373639,
-0.321859017169872));
#53579=CARTESIAN_POINT('Ctrl Pts',(-0.0566336279638654,0.020478815225617,
-0.31807488160688));
#53580=CARTESIAN_POINT('Ctrl Pts',(-0.0570163485729333,0.000825042249724007,
-0.316143001724741));
#53581=CARTESIAN_POINT('Ctrl Pts',(-0.0570135171869611,1.48812492774924E-5,
-0.316063377523455));
#53582=CARTESIAN_POINT('Ctrl Pts',(-0.0570093201057945,2.04236075452674E-5,
-0.344186622476545));
#53583=CARTESIAN_POINT('Ctrl Pts',(-0.0569273325535133,-0.0177002196552895,
-0.342445344849772));
#53584=CARTESIAN_POINT('Ctrl Pts',(-0.0385285285934815,-0.0544178041351661,
-0.338851811542146));
#53585=CARTESIAN_POINT('Ctrl Pts',(0.0239868036411113,-0.0628607521465771,
-0.333406022553666));
#53586=CARTESIAN_POINT('Ctrl Pts',(0.0658216455765284,-0.0139410144160481,
-0.327849255511104));
#53587=CARTESIAN_POINT('Ctrl Pts',(0.0474117200646131,0.0477385557999543,
-0.322292488468544));
#53588=CARTESIAN_POINT('Ctrl Pts',(-0.0143928672572947,0.0657243203195322,
-0.316735721425982));
#53589=CARTESIAN_POINT('Ctrl Pts',(-0.0526257584487598,0.032571147773634,
-0.31236709942865));
#53590=CARTESIAN_POINT('Ctrl Pts',(-0.056904254057181,0.00684303386737312,
-0.30985073311217));
#53591=CARTESIAN_POINT('Ctrl Pts',(-0.0568611677903335,3.91338492306548E-5,
-0.309186622476545));
#53592=CARTESIAN_POINT('Origin',(0.,0.,-0.648563377523455));
#53593=CARTESIAN_POINT('',(-0.0568360806176596,1.66360965570816E-5,-0.386063377523455));
#53594=CARTESIAN_POINT('',(-0.0569215673661572,-5.20456487798915E-5,-0.379186622476545));
#53595=CARTESIAN_POINT('',(-0.056925,-6.31153998696879E-15,-0.648563377523455));
#53596=CARTESIAN_POINT('Ctrl Pts',(-0.0568360806176596,1.66360965570813E-5,
-0.386063377523455));
#53597=CARTESIAN_POINT('Ctrl Pts',(-0.0568085040742901,-0.0105130658937851,
-0.385036736561652));
#53598=CARTESIAN_POINT('Ctrl Pts',(-0.0489531286766632,-0.0400785985646141,
-0.382157839918994));
#53599=CARTESIAN_POINT('Ctrl Pts',(-0.00136851012122178,-0.0672678843265587,
-0.377426687595484));
#53600=CARTESIAN_POINT('Ctrl Pts',(0.0557724726184293,-0.0376333944757582,
-0.371869920552923));
#53601=CARTESIAN_POINT('Ctrl Pts',(0.0618664234365842,0.0264459209122466,
-0.366313153510362));
#53602=CARTESIAN_POINT('Ctrl Pts',(0.0113357143866367,0.0663200019683107,
-0.360756386467801));
#53603=CARTESIAN_POINT('Ctrl Pts',(-0.0443802898012825,0.0472678976323277,
-0.355673127805499));
#53604=CARTESIAN_POINT('Ctrl Pts',(-0.056785527899603,0.0140417321827706,
-0.35244212482405));
#53605=CARTESIAN_POINT('Ctrl Pts',(-0.0569119761389687,-5.18431700991979E-5,
-0.351063377523455));
#53606=CARTESIAN_POINT('Ctrl Pts',(-0.0569215673661572,-5.2045648779895E-5,
-0.379186622476545));
#53607=CARTESIAN_POINT('Ctrl Pts',(-0.0569628786480138,-0.00456981308281385,
-0.378744467949081));
#53608=CARTESIAN_POINT('Ctrl Pts',(-0.0544066310307784,-0.0279670336518439,
-0.376450057740764));
#53609=CARTESIAN_POINT('Ctrl Pts',(-0.0221279122263006,-0.0635389361718822,
-0.372303391851593));
#53610=CARTESIAN_POINT('Ctrl Pts',(0.0413804763988367,-0.0530518339207716,
-0.366746624809032));
#53611=CARTESIAN_POINT('Ctrl Pts',(0.0670144370045379,0.00599217342164428,
-0.361189857766471));
#53612=CARTESIAN_POINT('Ctrl Pts',(0.031311900511308,0.0595517069085378,
-0.35563309072391));
#53613=CARTESIAN_POINT('Ctrl Pts',(-0.0330495695001504,0.0586051778020126,
-0.350076323681349));
#53614=CARTESIAN_POINT('Ctrl Pts',(-0.0564722426354389,0.0211241581890796,
-0.34626083426556));
#53615=CARTESIAN_POINT('Ctrl Pts',(-0.0570145454752997,0.00114982564897547,
-0.344297600530626));
#53616=CARTESIAN_POINT('Ctrl Pts',(-0.0570093201057945,2.04236075452674E-5,
-0.344186622476545));
#53617=CARTESIAN_POINT('Origin',(0.,0.,-0.648563377523455));
#53618=CARTESIAN_POINT('',(-0.0569729394550437,4.30825583782282E-5,-0.421063377523455));
#53619=CARTESIAN_POINT('',(-0.0568337016952294,1.15506553720647E-5,-0.414186622476544));
#53620=CARTESIAN_POINT('',(-0.056925,-6.31153998696879E-15,-0.648563377523455));
#53621=CARTESIAN_POINT('Ctrl Pts',(-0.0569729394550437,4.30825583782333E-5,
-0.421063377523455));
#53622=CARTESIAN_POINT('Ctrl Pts',(-0.0568374552814163,-0.0160609606593731,
-0.419483603980107));
#53623=CARTESIAN_POINT('Ctrl Pts',(-0.0412849050737077,-0.0512756220641729,
-0.416051574755906));
#53624=CARTESIAN_POINT('Ctrl Pts',(0.0184354247754988,-0.0647068481265139,
-0.41076728985085));
#53625=CARTESIAN_POINT('Ctrl Pts',(0.0643617662685185,-0.0196062266863109,
-0.40521052280829));
#53626=CARTESIAN_POINT('Ctrl Pts',(0.0513795282529356,0.0434394424251984,
-0.399653755765729));
#53627=CARTESIAN_POINT('Ctrl Pts',(-0.00862899881670666,0.0667261677385573,
-0.394096988723167));
#53628=CARTESIAN_POINT('Ctrl Pts',(-0.0511119318649797,0.0359213830672153,
-0.38956686264241));
#53629=CARTESIAN_POINT('Ctrl Pts',(-0.0568582574067744,0.00848452046303413,
-0.386888992242506));
#53630=CARTESIAN_POINT('Ctrl Pts',(-0.0568360806176596,1.66360965570813E-5,
-0.386063377523455));
#53631=CARTESIAN_POINT('Ctrl Pts',(-0.0568337016952294,1.1550655372063E-5,
-0.414186622476544));
#53632=CARTESIAN_POINT('Ctrl Pts',(-0.0568151834460149,-0.0101976377276981,
-0.413191335367536));
#53633=CARTESIAN_POINT('Ctrl Pts',(-0.0493106185827779,-0.0394317914459927,
-0.410343792577675));
#53634=CARTESIAN_POINT('Ctrl Pts',(-0.00250413919046523,-0.0672351857005294,
-0.40564399410696));
#53635=CARTESIAN_POINT('Ctrl Pts',(0.0551290772461912,-0.0385697517672564,
-0.400087227064398));
#53636=CARTESIAN_POINT('Ctrl Pts',(0.0623041440991956,0.0253975301438741,
-0.394530460021838));
#53637=CARTESIAN_POINT('Ctrl Pts',(0.0124539172307667,0.0661191413657922,
-0.388973692979276));
#53638=CARTESIAN_POINT('Ctrl Pts',(-0.0439214343045913,0.0478988281231328,
-0.383859080464179));
#53639=CARTESIAN_POINT('Ctrl Pts',(-0.056789819113961,0.0143558336644252,
-0.380596723629935));
#53640=CARTESIAN_POINT('Ctrl Pts',(-0.0569215673661572,-5.2045648779895E-5,
-0.379186622476545));
#53641=CARTESIAN_POINT('Origin',(0.,0.,-0.648563377523455));
#53642=CARTESIAN_POINT('',(-0.0569706330856471,-4.38941456312225E-5,-0.456063377523455));
#53643=CARTESIAN_POINT('',(-0.0569639325591123,4.59969122256296E-5,-0.449186622476545));
#53644=CARTESIAN_POINT('',(-0.056925,-6.31153998696879E-15,-0.648563377523455));
#53645=CARTESIAN_POINT('Ctrl Pts',(-0.0569706330856471,-4.38941456312194E-5,
-0.456063377523455));
#53646=CARTESIAN_POINT('Ctrl Pts',(-0.0569950085154664,-0.00290511617904001,
-0.455782727079417));
#53647=CARTESIAN_POINT('Ctrl Pts',(-0.0554983653945712,-0.0246244424230611,
-0.453649820954524));
#53648=CARTESIAN_POINT('Ctrl Pts',(-0.0275638766252995,-0.0613764922967096,
-0.449664659148778));
#53649=CARTESIAN_POINT('Ctrl Pts',(0.0366154427383043,-0.0564459954504943,
-0.444107892106218));
#53650=CARTESIAN_POINT('Ctrl Pts',(0.0672816408378267,0.000147989916712509,
-0.438551125063656));
#53651=CARTESIAN_POINT('Ctrl Pts',(0.03636677707249,0.0566065244349891,
-0.432994358021095));
#53652=CARTESIAN_POINT('Ctrl Pts',(-0.0278336114842633,0.0612546418564424,
-0.427437590978534));
#53653=CARTESIAN_POINT('Ctrl Pts',(-0.055549228542257,0.0244556428036377,
-0.42346059747932));
#53654=CARTESIAN_POINT('Ctrl Pts',(-0.0569963080051652,0.00282073644233923,
-0.421335859660961));
#53655=CARTESIAN_POINT('Ctrl Pts',(-0.0569729394550437,4.30825583782333E-5,
-0.421063377523455));
#53656=CARTESIAN_POINT('Ctrl Pts',(-0.0569639325591123,4.59969122256318E-5,
-0.449186622476545));
#53657=CARTESIAN_POINT('Ctrl Pts',(-0.0568253048831882,-0.0157449120098894,
-0.447638202785992));
#53658=CARTESIAN_POINT('Ctrl Pts',(-0.041791862645694,-0.0506568766499107,
-0.444237527414586));
#53659=CARTESIAN_POINT('Ctrl Pts',(0.0173402153203343,-0.0650089058319875,
-0.438984596362326));
#53660=CARTESIAN_POINT('Ctrl Pts',(0.0640215365519545,-0.0206901853312933,
-0.433427829319765));
#53661=CARTESIAN_POINT('Ctrl Pts',(0.0521056812744453,0.042565700843469,
-0.427871062277204));
#53662=CARTESIAN_POINT('Ctrl Pts',(-0.00750109120977298,0.0668623551738915,
-0.422314295234643));
#53663=CARTESIAN_POINT('Ctrl Pts',(-0.0507956988943071,0.0365710802835814,
-0.41775281530109));
#53664=CARTESIAN_POINT('Ctrl Pts',(-0.0568496463984601,0.00880193235444248,
-0.41504359104839));
#53665=CARTESIAN_POINT('Ctrl Pts',(-0.0568337016952294,1.1550655372063E-5,
-0.414186622476544));
#53666=CARTESIAN_POINT('Origin',(0.,0.,-0.648563377523455));
#53667=CARTESIAN_POINT('',(-0.0568353689804243,-1.53335310629876E-5,-0.491063377523455));
#53668=CARTESIAN_POINT('',(-0.0569793078036176,-4.05823445219014E-5,-0.484186622476545));
#53669=CARTESIAN_POINT('',(-0.056925,-6.31153998696879E-15,-0.648563377523455));
#53670=CARTESIAN_POINT('Ctrl Pts',(-0.0568353689804243,-1.53335310629811E-5,
-0.491063377523455));
#53671=CARTESIAN_POINT('Ctrl Pts',(-0.0568559923612236,-0.0085672539106082,
-0.490229594497872));
#53672=CARTESIAN_POINT('Ctrl Pts',(-0.0510302827578428,-0.0360906550071068,
-0.487543555791435));
#53673=CARTESIAN_POINT('Ctrl Pts',(-0.00833536402932787,-0.066763496614655,
-0.483005261404145));
#53674=CARTESIAN_POINT('Ctrl Pts',(0.0515701169003231,-0.0432129907282631,
-0.477448494361583));
#53675=CARTESIAN_POINT('Ctrl Pts',(0.064274898304406,0.019889166643205,
-0.471891727319023));
#53676=CARTESIAN_POINT('Ctrl Pts',(0.0181505921945029,0.06478732343249,
-0.466334960276461));
#53677=CARTESIAN_POINT('Ctrl Pts',(-0.041417849183696,0.0511146760956519,
-0.461058843677939));
#53678=CARTESIAN_POINT('Ctrl Pts',(-0.0568341339139286,0.0159785694809599,
-0.45763498276027));
#53679=CARTESIAN_POINT('Ctrl Pts',(-0.0569706330856471,-4.38941456312194E-5,
-0.456063377523455));
#53680=CARTESIAN_POINT('Ctrl Pts',(-0.0569793078036176,-4.05823445219027E-5,
-0.484186622476545));
#53681=CARTESIAN_POINT('Ctrl Pts',(-0.0569998081283525,-0.00258114455950157,
-0.483937325885302));
#53682=CARTESIAN_POINT('Ctrl Pts',(-0.0556913749191376,-0.0239766562237817,
-0.481835773613205));
#53683=CARTESIAN_POINT('Ctrl Pts',(-0.0285962923612928,-0.0609023247957534,
-0.477881965660254));
#53684=CARTESIAN_POINT('Ctrl Pts',(0.0356571255076543,-0.057056201086242,
-0.472325198617693));
#53685=CARTESIAN_POINT('Ctrl Pts',(0.0672745469504301,-0.000988088271253046,
-0.466768431575132));
#53686=CARTESIAN_POINT('Ctrl Pts',(0.0373173977562224,0.0559843974121422,
-0.461211664532571));
#53687=CARTESIAN_POINT('Ctrl Pts',(-0.0267953527133393,0.0617158808562009,
-0.45565489749001));
#53688=CARTESIAN_POINT('Ctrl Pts',(-0.0553517446039958,0.0251037241258535,
-0.451646550138001));
#53689=CARTESIAN_POINT('Ctrl Pts',(-0.0569911345363634,0.0031445408531103,
-0.449490458466846));
#53690=CARTESIAN_POINT('Ctrl Pts',(-0.0569639325591123,4.59969122256318E-5,
-0.449186622476545));
#53691=CARTESIAN_POINT('Origin',(0.,0.,-0.648563377523455));
#53692=CARTESIAN_POINT('',(-0.0569136073811911,5.1183173943782E-5,-0.526063377523456));
#53693=CARTESIAN_POINT('',(-0.0568383386836465,-2.03536804905466E-5,-0.519186622476545));
#53694=CARTESIAN_POINT('',(-0.056925,-6.31153998696879E-15,-0.648563377523455));
#53695=CARTESIAN_POINT('Ctrl Pts',(-0.0569136073811911,5.11831739437789E-5,
-0.526063377523456));
#53696=CARTESIAN_POINT('Ctrl Pts',(-0.0567858168353036,-0.0141241822318066,
-0.524676461916328));
#53697=CARTESIAN_POINT('Ctrl Pts',(-0.0442628394021531,-0.0474313237476093,
-0.521437290628346));
#53698=CARTESIAN_POINT('Ctrl Pts',(0.0116281096388898,-0.0662701761988158,
-0.516345863659512));
#53699=CARTESIAN_POINT('Ctrl Pts',(0.061981763895487,-0.0261731483262298,
-0.51078909661695));
#53700=CARTESIAN_POINT('Ctrl Pts',(0.0556065904708322,0.0378781889557639,
-0.505232329574389));
#53701=CARTESIAN_POINT('Ctrl Pts',(-0.00166452598691655,0.0672613134374671,
-0.499675562531828));
#53702=CARTESIAN_POINT('Ctrl Pts',(-0.0490469843264066,0.0399101343193825,
-0.49495257851485));
#53703=CARTESIAN_POINT('Ctrl Pts',(-0.0568101773553145,0.0104309058254248,
-0.492081850178726));
#53704=CARTESIAN_POINT('Ctrl Pts',(-0.0568353689804243,-1.53335310629811E-5,
-0.491063377523455));
#53705=CARTESIAN_POINT('Ctrl Pts',(-0.0568383386836465,-2.03536804905492E-5,
-0.519186622476545));
#53706=CARTESIAN_POINT('Ctrl Pts',(-0.0568647265358007,-0.00824955685581068,
-0.518384193303757));
#53707=CARTESIAN_POINT('Ctrl Pts',(-0.0513411570398651,-0.0354405810816032,
-0.515729508450115));
#53708=CARTESIAN_POINT('Ctrl Pts',(-0.00946140608284985,-0.066613336227403,
-0.511222567915621));
#53709=CARTESIAN_POINT('Ctrl Pts',(0.0508330680958483,-0.0440775413718835,
-0.505665800873059));
#53710=CARTESIAN_POINT('Ctrl Pts',(0.0646015856194826,0.0188010149829039,
-0.500109033830499));
#53711=CARTESIAN_POINT('Ctrl Pts',(0.0192419326369567,0.0644716265578821,
-0.494552266787937));
#53712=CARTESIAN_POINT('Ctrl Pts',(-0.0409041756051557,0.0517314628965133,
-0.48924479633662));
#53713=CARTESIAN_POINT('Ctrl Pts',(-0.0568474921951092,0.0162950493418725,
-0.485789581566155));
#53714=CARTESIAN_POINT('Ctrl Pts',(-0.0569793078036176,-4.05823445219027E-5,
-0.484186622476545));
#53715=CARTESIAN_POINT('Origin',(0.,0.,-0.648563377523455));
#53716=CARTESIAN_POINT('',(-0.056925,-6.31153998696879E-15,-0.5608));
#53717=CARTESIAN_POINT('',(-0.0569002140125902,4.52833130624476E-5,-0.554186622476545));
#53718=CARTESIAN_POINT('',(-0.056925,-6.31153998696879E-15,-0.648563377523455));
#53719=CARTESIAN_POINT('',(-0.0568613829974076,-0.00269049226390444,-0.5608));
#53720=CARTESIAN_POINT('Origin',(0.,0.,-0.5608));
#53721=CARTESIAN_POINT('Ctrl Pts',(-0.0568613829974076,-0.00269049226390446,
-0.5608));
#53722=CARTESIAN_POINT('Ctrl Pts',(-0.0559667508352254,-0.0215978211189658,
-0.558947744319147));
#53723=CARTESIAN_POINT('Ctrl Pts',(-0.033852782438917,-0.0581229253359501,
-0.555243232957439));
#53724=CARTESIAN_POINT('Ctrl Pts',(0.0306018951616518,-0.0599703320683201,
-0.549686465914878));
#53725=CARTESIAN_POINT('Ctrl Pts',(0.0669157535097345,-0.00681168427321597,
-0.544129698872316));
#53726=CARTESIAN_POINT('Ctrl Pts',(0.0420494689529653,0.0525221733225254,
-0.538572931829757));
#53727=CARTESIAN_POINT('Ctrl Pts',(-0.0213379694595951,0.0638149374263822,
-0.533016164787193));
#53728=CARTESIAN_POINT('Ctrl Pts',(-0.0542353794736302,0.0284468929477895,
-0.528846313351762));
#53729=CARTESIAN_POINT('Ctrl Pts',(-0.0569564838631769,0.00480732374162209,
-0.526528717597182));
#53730=CARTESIAN_POINT('Ctrl Pts',(-0.0569136073811911,5.11831739437789E-5,
-0.526063377523456));
#53731=CARTESIAN_POINT('Ctrl Pts',(-0.0569002140125902,4.52833130624433E-5,
-0.554186622476545));
#53732=CARTESIAN_POINT('Ctrl Pts',(-0.0567793059135598,-0.0138144038624156,
-0.552831060722212));
#53733=CARTESIAN_POINT('Ctrl Pts',(-0.0447210948641033,-0.046791207995725,
-0.549623243287027));
#53734=CARTESIAN_POINT('Ctrl Pts',(0.0105110504745919,-0.0664618166825911,
-0.544563170170987));
#53735=CARTESIAN_POINT('Ctrl Pts',(0.0615291043141801,-0.0272134801016605,
-0.539006403128426));
#53736=CARTESIAN_POINT('Ctrl Pts',(0.0562392334272427,0.0369325451809627,
-0.533449636085865));
#53737=CARTESIAN_POINT('Ctrl Pts',(-0.000529100216082706,0.0672805255553111,
-0.527892869043304));
#53738=CARTESIAN_POINT('Ctrl Pts',(-0.048683516574914,0.0405561571276554,
-0.52313853117353));
#53739=CARTESIAN_POINT('Ctrl Pts',(-0.0568038151797388,0.0107459991973579,
-0.520236448984611));
#53740=CARTESIAN_POINT('Ctrl Pts',(-0.0568383386836465,-2.03536804905492E-5,
-0.519186622476545));
#53741=CARTESIAN_POINT('Ctrl Pts',(0.0565254421840275,-0.00673275656029218,
-0.572347005383793));
#53742=CARTESIAN_POINT('Ctrl Pts',(0.0587641925568829,0.0120628665447577,
-0.570494749702939));
#53743=CARTESIAN_POINT('Ctrl Pts',(0.04298296994418,0.0517373268281049,
-0.566790238341231));
#53744=CARTESIAN_POINT('Ctrl Pts',(-0.0202825412718916,0.0641991901194383,
-0.561233471298671));
#53745=CARTESIAN_POINT('Ctrl Pts',(-0.06487330649251,0.0177642870332536,
-0.555676704256109));
#53746=CARTESIAN_POINT('Ctrl Pts',(-0.0501426511359929,-0.0448603521282914,
-0.550119937213548));
#53747=CARTESIAN_POINT('Ctrl Pts',(0.0105110504745919,-0.0664618166825911,
-0.544563170170987));
#53748=CARTESIAN_POINT('Ctrl Pts',(0.0615291043141801,-0.0272134801016605,
-0.539006403128426));
#53749=CARTESIAN_POINT('Ctrl Pts',(0.0562392334272427,0.0369325451809627,
-0.533449636085865));
#53750=CARTESIAN_POINT('Ctrl Pts',(-0.000529100216082706,0.0672805255553111,
-0.527892869043304));
#53751=CARTESIAN_POINT('Ctrl Pts',(-0.0568109382145401,0.0360456630403476,
-0.522336102000743));
#53752=CARTESIAN_POINT('Ctrl Pts',(-0.0610964383375367,-0.0281793393520896,
-0.516779334958181));
#53753=CARTESIAN_POINT('Ctrl Pts',(-0.00946140608284985,-0.066613336227403,
-0.511222567915621));
#53754=CARTESIAN_POINT('Ctrl Pts',(0.0508330680958483,-0.0440775413718835,
-0.505665800873059));
#53755=CARTESIAN_POINT('Ctrl Pts',(0.0646015856194826,0.0188010149829039,
-0.500109033830499));
#53756=CARTESIAN_POINT('Ctrl Pts',(0.0192419326369567,0.0644716265578821,
-0.494552266787937));
#53757=CARTESIAN_POINT('Ctrl Pts',(-0.0437292916182991,0.0511330461174107,
-0.488995499745377));
#53758=CARTESIAN_POINT('Ctrl Pts',(-0.0666763062528489,-0.00900619312042977,
-0.483438732702815));
#53759=CARTESIAN_POINT('Ctrl Pts',(-0.0285962923612928,-0.0609023247957534,
-0.477881965660254));
#53760=CARTESIAN_POINT('Ctrl Pts',(0.0356571255076543,-0.057056201086242,
-0.472325198617693));
#53761=CARTESIAN_POINT('Ctrl Pts',(0.0672745469504301,-0.000988088271253046,
-0.466768431575132));
#53762=CARTESIAN_POINT('Ctrl Pts',(0.0373173977562224,0.0559843974121422,
-0.461211664532571));
#53763=CARTESIAN_POINT('Ctrl Pts',(-0.0267953527133393,0.0617158808562009,
-0.45565489749001));
#53764=CARTESIAN_POINT('Ctrl Pts',(-0.0663830439429782,0.0109604926600342,
-0.450098130447448));
#53765=CARTESIAN_POINT('Ctrl Pts',(-0.0452121347354353,-0.0498267376368557,
-0.444541363404887));
#53766=CARTESIAN_POINT('Ctrl Pts',(0.0173402153203343,-0.0650089058319875,
-0.438984596362326));
#53767=CARTESIAN_POINT('Ctrl Pts',(0.0640215365519545,-0.0206901853312933,
-0.433427829319765));
#53768=CARTESIAN_POINT('Ctrl Pts',(0.0521056812744453,0.042565700843469,
-0.427871062277204));
#53769=CARTESIAN_POINT('Ctrl Pts',(-0.00750109120977298,0.0668623551738915,
-0.422314295234643));
#53770=CARTESIAN_POINT('Ctrl Pts',(-0.0602423183129323,0.0299617087960569,
-0.416757528192082));
#53771=CARTESIAN_POINT('Ctrl Pts',(-0.0578453849239086,-0.034362077241173,
-0.411200761149521));
#53772=CARTESIAN_POINT('Ctrl Pts',(-0.00250413919046523,-0.0672351857005294,
-0.40564399410696));
#53773=CARTESIAN_POINT('Ctrl Pts',(0.0551290772461912,-0.0385697517672564,
-0.400087227064398));
#53774=CARTESIAN_POINT('Ctrl Pts',(0.0623041440991956,0.0253975301438741,
-0.394530460021838));
#53775=CARTESIAN_POINT('Ctrl Pts',(0.0124539172307667,0.0661191413657922,
-0.388973692979276));
#53776=CARTESIAN_POINT('Ctrl Pts',(-0.0487950423922266,0.0463236953113581,
-0.383416925936716));
#53777=CARTESIAN_POINT('Ctrl Pts',(-0.0653832227873078,-0.0158705729982893,
-0.377860158894154));
#53778=CARTESIAN_POINT('Ctrl Pts',(-0.0221279122263006,-0.0635389361718822,
-0.372303391851593));
#53779=CARTESIAN_POINT('Ctrl Pts',(0.0413804763988367,-0.0530518339207716,
-0.366746624809032));
#53780=CARTESIAN_POINT('Ctrl Pts',(0.0670144370045379,0.00599217342164428,
-0.361189857766471));
#53781=CARTESIAN_POINT('Ctrl Pts',(0.031311900511308,0.0595517069085378,
-0.35563309072391));
#53782=CARTESIAN_POINT('Ctrl Pts',(-0.0330495695001504,0.0586051778020126,
-0.350076323681349));
#53783=CARTESIAN_POINT('Ctrl Pts',(-0.0671616646846567,0.00401891852819577,
-0.344519556638788));
#53784=CARTESIAN_POINT('Ctrl Pts',(-0.0398025092666771,-0.0542457479018093,
-0.338962789596227));
#53785=CARTESIAN_POINT('Ctrl Pts',(0.0239868036411113,-0.0628607521465771,
-0.333406022553666));
#53786=CARTESIAN_POINT('Ctrl Pts',(0.0658216455765284,-0.0139410144160481,
-0.327849255511104));
#53787=CARTESIAN_POINT('Ctrl Pts',(0.0474117200646131,0.0477385557999543,
-0.322292488468544));
#53788=CARTESIAN_POINT('Ctrl Pts',(-0.0143928672572947,0.0657243203195322,
-0.316735721425982));
#53789=CARTESIAN_POINT('Ctrl Pts',(-0.063024053440091,0.0235543965605395,
-0.311178954383422));
#53790=CARTESIAN_POINT('Ctrl Pts',(-0.0539710324015399,-0.0401742276946618,
-0.30562218734086));
#53791=CARTESIAN_POINT('Ctrl Pts',(0.00448021117374274,-0.0671324706620369,
-0.300065420298299));
#53792=CARTESIAN_POINT('Ctrl Pts',(0.0588308389422806,-0.0326461835242353,
-0.294508653255737));
#53793=CARTESIAN_POINT('Ctrl Pts',(0.0593351950206278,0.0317202701945406,
-0.288951886213177));
#53794=CARTESIAN_POINT('Ctrl Pts',(0.00553165596584969,0.067054020696943,
-0.283395119170615));
#53795=CARTESIAN_POINT('Ctrl Pts',(-0.0533348578040438,0.0410150442200543,
-0.277838352128055));
#53796=CARTESIAN_POINT('Ctrl Pts',(-0.063385422396469,-0.0225638901116765,
-0.272281585085493));
#53797=CARTESIAN_POINT('Ctrl Pts',(-0.0154210285602653,-0.0654907076423372,
-0.266724818042933));
#53798=CARTESIAN_POINT('Ctrl Pts',(0.0466578145771441,-0.0484756562434736,
-0.261168051000371));
#53799=CARTESIAN_POINT('Ctrl Pts',(0.0660320251551521,0.0129078489013458,
-0.255611283957811));
#53800=CARTESIAN_POINT('Ctrl Pts',(0.024968913561939,0.062477149942095,
-0.250054516915249));
#53801=CARTESIAN_POINT('Ctrl Pts',(-0.0389475675843432,0.0548628097039661,
-0.244497749872688));
#53802=CARTESIAN_POINT('Ctrl Pts',(-0.0672163961809798,-0.00296597265533152,
-0.238940982830127));
#53803=CARTESIAN_POINT('Ctrl Pts',(-0.0339638799205846,-0.0580800806653254,
-0.233384215787566));
#53804=CARTESIAN_POINT('Ctrl Pts',(0.0303748547031255,-0.0600350656792724,
-0.227827448745005));
#53805=CARTESIAN_POINT('Ctrl Pts',(0.066912308428919,-0.00704158292317649,
-0.222270681702444));
#53806=CARTESIAN_POINT('Ctrl Pts',(0.0422067405718221,0.0523968697505238,
-0.216713914659883));
#53807=CARTESIAN_POINT('Ctrl Pts',(-0.0211295124981265,0.0638778882786663,
-0.211157147617322));
#53808=CARTESIAN_POINT('Ctrl Pts',(-0.0651264957036645,0.0168932077093837,
-0.20560038057476));
#53809=CARTESIAN_POINT('Ctrl Pts',(-0.0495149632915362,-0.0455533678182764,
-0.2000436135322));
#53810=CARTESIAN_POINT('Ctrl Pts',(0.0114162724268508,-0.0663061809579219,
-0.194486846489638));
#53811=CARTESIAN_POINT('Ctrl Pts',(0.0618985035444009,-0.0263707445538147,
-0.188930079447077));
#53812=CARTESIAN_POINT('Ctrl Pts',(0.0557267127407225,0.0377011192997421,
-0.183373312404516));
#53813=CARTESIAN_POINT('Ctrl Pts',(-0.00145022720861101,0.067266170921093,
-0.177816545361955));
#53814=CARTESIAN_POINT('Ctrl Pts',(-0.0572998135174467,0.0352643202156253,
-0.172259778319394));
#53815=CARTESIAN_POINT('Ctrl Pts',(-0.0607044341923943,-0.0290140065942496,
-0.166703011276833));
#53816=CARTESIAN_POINT('Ctrl Pts',(-0.00854793224978894,-0.0667365998802494,
-0.161146244234271));
#53817=CARTESIAN_POINT('Ctrl Pts',(0.0514322603095934,-0.0433769928549986,
-0.155589477191711));
#53818=CARTESIAN_POINT('Ctrl Pts',(0.0643378995797782,0.019684399569185,
-0.150032710149149));
#53819=CARTESIAN_POINT('Ctrl Pts',(0.0183568039000239,0.0647291948037812,
-0.144475943106589));
#53820=CARTESIAN_POINT('Ctrl Pts',(-0.0444257766806479,0.0505291131709007,
-0.138919176064027));
#53821=CARTESIAN_POINT('Ctrl Pts',(-0.0665466484015406,-0.00991889567187386,
-0.133362409021467));
#53822=CARTESIAN_POINT('Ctrl Pts',(-0.0277591773719423,-0.0612884082229279,
-0.127805641978905));
#53823=CARTESIAN_POINT('Ctrl Pts',(0.0364355162536436,-0.0565623026212381,
-0.122248874936344));
#53824=CARTESIAN_POINT('Ctrl Pts',(0.0672817693522171,-6.62549929698068E-5,
-0.116692107893783));
#53825=CARTESIAN_POINT('Ctrl Pts',(0.0365468441487368,0.0564904338066607,
-0.111135340851222));
#53826=CARTESIAN_POINT('Ctrl Pts',(-0.0276384181430455,0.0613429607075467,
-0.105578573808661));
#53827=CARTESIAN_POINT('Ctrl Pts',(-0.0665269826816367,0.0100499381659545,
-0.1000218067661));
#53828=CARTESIAN_POINT('Ctrl Pts',(-0.044525209609633,-0.0504415187277128,
-0.0944650397235386));
#53829=CARTESIAN_POINT('Ctrl Pts',(0.0182292914472235,-0.0647652241822597,
-0.0889082726809775));
#53830=CARTESIAN_POINT('Ctrl Pts',(0.0642989956139634,-0.0198110704839244,
-0.0833515056384163));
#53831=CARTESIAN_POINT('Ctrl Pts',(0.0515176118264206,0.0432756083068328,
-0.0777947385958553));
#53832=CARTESIAN_POINT('Ctrl Pts',(-0.00841651961310768,0.0667533162213003,
-0.0722379715532942));
#53833=CARTESIAN_POINT('Ctrl Pts',(-0.0606470977391485,0.0291334859096097,
-0.0666812045107331));
#53834=CARTESIAN_POINT('Ctrl Pts',(-0.0573692992813992,-0.0351513622548381,
-0.0611244374681719));
#53835=CARTESIAN_POINT('Ctrl Pts',(-0.00158242957906591,-0.0672632578788742,
-0.055567670425611));
#53836=CARTESIAN_POINT('Ctrl Pts',(0.0556518335368746,-0.0378106591957688,
-0.0500109033830497));
#53837=CARTESIAN_POINT('Ctrl Pts',(0.0619513051118907,0.0262485211196931,
-0.0444541363404888));
#53838=CARTESIAN_POINT('Ctrl Pts',(0.0115449715450025,0.0662840697456999,
-0.0388973692979276));
#53839=CARTESIAN_POINT('Ctrl Pts',(-0.0494216107805867,0.0456498473688679,
-0.0333406022553666));
#53840=CARTESIAN_POINT('Ctrl Pts',(-0.0651663525864486,-0.0167631067946381,
-0.0277838352128054));
#53841=CARTESIAN_POINT('Ctrl Pts',(-0.0212425420460525,-0.0638395728638739,
-0.0222270681702444));
#53842=CARTESIAN_POINT('Ctrl Pts',(0.0420792312090032,-0.0524733655289061,
-0.0166703011276832));
#53843=CARTESIAN_POINT('Ctrl Pts',(0.0669727390520183,0.00689708027414815,
-0.0111135340851222));
#53844=CARTESIAN_POINT('Ctrl Pts',(0.0303982238704425,0.0600019556186538,
-0.00555676704256101));
#53845=CARTESIAN_POINT('Ctrl Pts',(-0.012280390439628,0.0587191202828289,
-0.00185225568085369));
#53846=CARTESIAN_POINT('Ctrl Pts',(-0.0286389268003753,0.0491962142519396,
0.));
#53847=CARTESIAN_POINT('Ctrl Pts',(0.0631453153720266,-0.00752125096056136,
-0.568498003589195));
#53848=CARTESIAN_POINT('Ctrl Pts',(0.0656462528768225,0.013475586971606,
-0.566645747908341));
#53849=CARTESIAN_POINT('Ctrl Pts',(0.0480168414059497,0.057796448693495,
-0.562941236546634));
#53850=CARTESIAN_POINT('Ctrl Pts',(-0.022657893785068,0.0717177601817357,
-0.557384469504073));
#53851=CARTESIAN_POINT('Ctrl Pts',(-0.0724708244538636,0.0198447188333718,
-0.551827702461512));
#53852=CARTESIAN_POINT('Ctrl Pts',(-0.0560150154909626,-0.0501140897512789,
-0.54627093541895));
#53853=CARTESIAN_POINT('Ctrl Pts',(0.0117420328168065,-0.0742453700929372,
-0.54071416837639));
#53854=CARTESIAN_POINT('Ctrl Pts',(0.0687349721887727,-0.0304005367670585,
-0.535157401333827));
#53855=CARTESIAN_POINT('Ctrl Pts',(0.0628255878031463,0.04125783227579,
-0.529600634291268));
#53856=CARTESIAN_POINT('Ctrl Pts',(-0.00059106481465686,0.0751599605493455,
-0.524043867248705));
#53857=CARTESIAN_POINT('Ctrl Pts',(-0.0634642467450084,0.0402670845646169,
-0.518487100206145));
#53858=CARTESIAN_POINT('Ctrl Pts',(-0.0682516353321248,-0.0314795108469903,
-0.512930333163584));
#53859=CARTESIAN_POINT('Ctrl Pts',(-0.0105694612528521,-0.0744146345705331,
-0.507373566121023));
#53860=CARTESIAN_POINT('Ctrl Pts',(0.0567862893631114,-0.0492396015530446,
-0.501816799078462));
#53861=CARTESIAN_POINT('Ctrl Pts',(0.0721672814905979,0.0210028612698777,
-0.496260032035901));
#53862=CARTESIAN_POINT('Ctrl Pts',(0.0214954161839588,0.0720221025125452,
-0.49070326499334));
#53863=CARTESIAN_POINT('Ctrl Pts',(-0.0488505671701414,0.0571213987588882,
-0.485146497950779));
#53864=CARTESIAN_POINT('Ctrl Pts',(-0.0744849792146817,-0.0100609368616591,
-0.479589730908218));
#53865=CARTESIAN_POINT('Ctrl Pts',(-0.031945294540921,-0.0680347885399491,
-0.474032963865656));
#53866=CARTESIAN_POINT('Ctrl Pts',(0.03983304417346,-0.063738233126792,
-0.468476196823096));
#53867=CARTESIAN_POINT('Ctrl Pts',(0.075153281771151,-0.00110380641164368,
-0.462919429780533));
#53868=CARTESIAN_POINT('Ctrl Pts',(0.0416877561525016,0.0625409071368838,
-0.457362662737974));
#53869=CARTESIAN_POINT('Ctrl Pts',(-0.0299334411587596,0.0689436227219545,
-0.451805895695412));
#53870=CARTESIAN_POINT('Ctrl Pts',(-0.0741573720288194,0.0122441105970908,
-0.446249128652851));
#53871=CARTESIAN_POINT('Ctrl Pts',(-0.0505070707313879,-0.0556621043634669,
-0.44069236161029));
#53872=CARTESIAN_POINT('Ctrl Pts',(0.0193709827418336,-0.0726223042605618,
-0.435135594567729));
#53873=CARTESIAN_POINT('Ctrl Pts',(0.0715193010434728,-0.0231132783286642,
-0.429578827525168));
#53874=CARTESIAN_POINT('Ctrl Pts',(0.0582079422932654,0.047550704602036,
-0.424022060482607));
#53875=CARTESIAN_POINT('Ctrl Pts',(-0.00837956770923311,0.0746928169128921,
-0.418465293440046));
#53876=CARTESIAN_POINT('Ctrl Pts',(-0.067297486611914,0.0334706192098838,
-0.412908526397484));
#53877=CARTESIAN_POINT('Ctrl Pts',(-0.0646198407779753,-0.0383863287113727,
-0.407351759354924));
#53878=CARTESIAN_POINT('Ctrl Pts',(-0.00279740684562234,-0.0751093108008694,
-0.401794992312362));
#53879=CARTESIAN_POINT('Ctrl Pts',(0.0615854177229808,-0.0430867772999472,
-0.396238225269801));
#53880=CARTESIAN_POINT('Ctrl Pts',(0.069600779332596,0.0283719151702384,
-0.39068145822724));
#53881=CARTESIAN_POINT('Ctrl Pts',(0.0139124348394066,0.0738625629867309,
-0.385124691184679));
#53882=CARTESIAN_POINT('Ctrl Pts',(-0.054509584027972,0.051748809679546,
-0.379567924142117));
#53883=CARTESIAN_POINT('Ctrl Pts',(-0.0730404586575827,-0.0177292259625151,
-0.374011157099557));
#53884=CARTESIAN_POINT('Ctrl Pts',(-0.024719381964413,-0.0709801818075876,
-0.368454390056995));
#53885=CARTESIAN_POINT('Ctrl Pts',(0.0462266747766825,-0.0592649018664049,
-0.362897623014435));
#53886=CARTESIAN_POINT('Ctrl Pts',(0.0748627095273941,0.00669393578986403,
-0.357340855971873));
#53887=CARTESIAN_POINT('Ctrl Pts',(0.0349789361443122,0.0665259955232103,
-0.351784088929313));
#53888=CARTESIAN_POINT('Ctrl Pts',(-0.0369201090404981,0.0654686154014289,
-0.346227321886751));
#53889=CARTESIAN_POINT('Ctrl Pts',(-0.0750271795064581,0.00448958677919307,
-0.34067055484419));
#53890=CARTESIAN_POINT('Ctrl Pts',(-0.0444639069263677,-0.0605986388872351,
-0.335113787801629));
#53891=CARTESIAN_POINT('Ctrl Pts',(0.0267959740280068,-0.0702225735076171,
-0.329557020759068));
#53892=CARTESIAN_POINT('Ctrl Pts',(0.0735302265253239,-0.0155736906761628,
-0.324000253716507));
#53893=CARTESIAN_POINT('Ctrl Pts',(0.0529642564504562,0.0533293689517563,
-0.318443486673946));
#53894=CARTESIAN_POINT('Ctrl Pts',(-0.0160784614317684,0.0734215031998758,
-0.312886719631385));
#53895=CARTESIAN_POINT('Ctrl Pts',(-0.0704049995317425,0.0263129263875688,
-0.307329952588823));
#53896=CARTESIAN_POINT('Ctrl Pts',(-0.0602917505864667,-0.0448791584743024,
-0.301773185546263));
#53897=CARTESIAN_POINT('Ctrl Pts',(0.00500490286441585,-0.074994566479579,
-0.296216418503701));
#53898=CARTESIAN_POINT('Ctrl Pts',(0.0657207044310556,-0.0364694812580068,
-0.290659651461141));
#53899=CARTESIAN_POINT('Ctrl Pts',(0.0662841272438023,0.0354351312918364,
-0.285102884418579));
#53900=CARTESIAN_POINT('Ctrl Pts',(0.00617948567931561,0.0749069289911245,
-0.279546117376018));
#53901=CARTESIAN_POINT('Ctrl Pts',(-0.0595810715711688,0.0458184456804626,
-0.273989350333457));
#53902=CARTESIAN_POINT('Ctrl Pts',(-0.070808689548742,-0.0252064185978917,
-0.268432583290896));
#53903=CARTESIAN_POINT('Ctrl Pts',(-0.0172270339545294,-0.0731605314036999,
-0.262875816248335));
#53904=CARTESIAN_POINT('Ctrl Pts',(0.0521220587085613,-0.0541527935578907,
-0.257319049205774));
#53905=CARTESIAN_POINT('Ctrl Pts',(0.0737652443213244,0.014419527882618,
-0.251762282163213));
#53906=CARTESIAN_POINT('Ctrl Pts',(0.0278931019457125,0.0697940464365575,
-0.246205515120652));
#53907=CARTESIAN_POINT('Ctrl Pts',(-0.0435088403214929,0.0612879667473238,
-0.240648748078091));
#53908=CARTESIAN_POINT('Ctrl Pts',(-0.0750883207812995,-0.00331332708722427,
-0.235091981035529));
#53909=CARTESIAN_POINT('Ctrl Pts',(-0.0379414972440325,-0.0648820224794459,
-0.229535213992968));
#53910=CARTESIAN_POINT('Ctrl Pts',(0.0339321499399129,-0.067065961967286,
-0.223978446950407));
#53911=CARTESIAN_POINT('Ctrl Pts',(0.0747486203514977,-0.00786624495487712,
-0.218421679907846));
#53912=CARTESIAN_POINT('Ctrl Pts',(0.047149705358451,0.0585332327721041,
-0.212864912865285));
#53913=CARTESIAN_POINT('Ctrl Pts',(-0.0236040564885372,0.0713588296668868,
-0.207308145822724));
#53914=CARTESIAN_POINT('Ctrl Pts',(-0.0727536654537641,0.0188716246567578,
-0.201751378780163));
#53915=CARTESIAN_POINT('Ctrl Pts',(-0.0553138171391768,-0.0508882666990576,
-0.196194611737602));
#53916=CARTESIAN_POINT('Ctrl Pts',(0.0127532681729312,-0.0740715073766511,
-0.190637844695041));
#53917=CARTESIAN_POINT('Ctrl Pts',(0.0691476329303646,-0.0294591057956617,
-0.18508107765248));
#53918=CARTESIAN_POINT('Ctrl Pts',(0.0622530441991593,0.0421164165387684,
-0.179524310609919));
#53919=CARTESIAN_POINT('Ctrl Pts',(-0.00162006790058625,0.0751439247985451,
-0.173967543567357));
#53920=CARTESIAN_POINT('Ctrl Pts',(-0.0640103757797735,0.0393942362121858,
-0.168410776524797));
#53921=CARTESIAN_POINT('Ctrl Pts',(-0.06781372234258,-0.0324119286079217,
-0.162854009482235));
#53922=CARTESIAN_POINT('Ctrl Pts',(-0.00954900761208391,-0.0745523340193503,
-0.157297242439674));
#53923=CARTESIAN_POINT('Ctrl Pts',(0.05745565487081,-0.0484570095851997,
-0.151740475397113));
#53924=CARTESIAN_POINT('Ctrl Pts',(0.0718727143453798,0.0219897018170759,
-0.146183708354552));
#53925=CARTESIAN_POINT('Ctrl Pts',(0.0205066272231135,0.0723098353897895,
-0.140626941311991));
#53926=CARTESIAN_POINT('Ctrl Pts',(-0.0496286197994466,0.0564467373162272,
-0.13507017426943));
#53927=CARTESIAN_POINT('Ctrl Pts',(-0.0743401367226111,-0.0110805288935828,
-0.129513407226869));
#53928=CARTESIAN_POINT('Ctrl Pts',(-0.0310101423693891,-0.0684660874175319,
-0.123956640184308));
#53929=CARTESIAN_POINT('Ctrl Pts',(0.0407025947198872,-0.0631864926515402,
-0.118399873141746));
#53930=CARTESIAN_POINT('Ctrl Pts',(0.0751613500112382,-7.40143246023484E-5,
-0.112843106099186));
#53931=CARTESIAN_POINT('Ctrl Pts',(0.0408269605766383,0.0631062070529388,
-0.107286339056624));
#53932=CARTESIAN_POINT('Ctrl Pts',(-0.030875240645524,0.0685270287160431,
-0.101729572014063));
#53933=CARTESIAN_POINT('Ctrl Pts',(-0.0743181678880937,0.0112269181883187,
-0.0961728049715021));
#53934=CARTESIAN_POINT('Ctrl Pts',(-0.0497396976330133,-0.0563488844109461,
-0.090616037928941));
#53935=CARTESIAN_POINT('Ctrl Pts',(0.0203641813839491,-0.0723500842826564,
-0.08505927088638));
#53936=CARTESIAN_POINT('Ctrl Pts',(0.0718292542131685,-0.022131207562997,
-0.0795025038438188));
#53937=CARTESIAN_POINT('Ctrl Pts',(0.0575510021735351,0.0483437515721617,
-0.0739457368012578));
#53938=CARTESIAN_POINT('Ctrl Pts',(-0.00940220482617748,0.0745710080639356,
-0.0683889697586965));
#53939=CARTESIAN_POINT('Ctrl Pts',(-0.0677496710360767,0.0325454005235305,
-0.0628322027161357));
#53940=CARTESIAN_POINT('Ctrl Pts',(-0.0640879992411595,-0.0392680493875954,
-0.0572754356735743));
#53941=CARTESIAN_POINT('Ctrl Pts',(-0.00176775290848452,-0.0751406706007451,
-0.0517186686310135));
#53942=CARTESIAN_POINT('Ctrl Pts',(0.0621693956550852,-0.0422387849982311,
-0.0461619015884522));
#53943=CARTESIAN_POINT('Ctrl Pts',(0.069206618256308,0.0293225683888702,
-0.0406051345458912));
#53944=CARTESIAN_POINT('Ctrl Pts',(0.0128970396515766,0.074046806650481,
-0.0350483675033301));
#53945=CARTESIAN_POINT('Ctrl Pts',(-0.0552095318206196,0.0509960452747527,
-0.029491600460769));
#53946=CARTESIAN_POINT('Ctrl Pts',(-0.0727981901020628,-0.0187262872126889,
-0.0239348334182079));
#53947=CARTESIAN_POINT('Ctrl Pts',(-0.0237303232840627,-0.0713160270127682,
-0.0183780663756468));
#53948=CARTESIAN_POINT('Ctrl Pts',(0.0470072629711461,-0.0586186872128659,
-0.0128212993330857));
#53949=CARTESIAN_POINT('Ctrl Pts',(0.0748161281958647,0.00770481914390555,
-0.00726453229052467));
#53950=CARTESIAN_POINT('Ctrl Pts',(0.0339582559442764,0.0670289742828201,
-0.00170776524796349));
#53951=CARTESIAN_POINT('Ctrl Pts',(-0.0137185857773087,0.065595902046299,
0.00199674611374385));
#53952=CARTESIAN_POINT('Ctrl Pts',(-0.031992922033913,0.0549577383921174,
0.00384900179459754));
#53953=CARTESIAN_POINT('Ctrl Pts',(0.0697651885600256,-0.00830974536083054,
-0.564649001794598));
#53954=CARTESIAN_POINT('Ctrl Pts',(0.0725283131967621,0.0148883073984543,
-0.562796746113744));
#53955=CARTESIAN_POINT('Ctrl Pts',(0.0530507128677194,0.0638555705588852,
-0.559092234752036));
#53956=CARTESIAN_POINT('Ctrl Pts',(-0.0250332462982443,0.0792363302440328,
-0.553535467709476));
#53957=CARTESIAN_POINT('Ctrl Pts',(-0.0800683424152172,0.0219251506334903,
-0.547978700666914));
#53958=CARTESIAN_POINT('Ctrl Pts',(-0.0618873798459324,-0.0553678273742666,
-0.542421933624354));
#53959=CARTESIAN_POINT('Ctrl Pts',(0.0129730151590211,-0.0820289235032833,
-0.536865166581792));
#53960=CARTESIAN_POINT('Ctrl Pts',(0.0759408400633652,-0.0335875934324565,
-0.53130839953923));
#53961=CARTESIAN_POINT('Ctrl Pts',(0.0694119421790499,0.0455831193706172,
-0.525751632496671));
#53962=CARTESIAN_POINT('Ctrl Pts',(-0.000653029413231036,0.08303939554338,
-0.520194865454108));
#53963=CARTESIAN_POINT('Ctrl Pts',(-0.0701175552754767,0.044488506088886,
-0.514638098411548));
#53964=CARTESIAN_POINT('Ctrl Pts',(-0.0754068323267131,-0.0347796823418909,
-0.509081331368986));
#53965=CARTESIAN_POINT('Ctrl Pts',(-0.0116775164228544,-0.0822159329136632,
-0.503524564326426));
#53966=CARTESIAN_POINT('Ctrl Pts',(0.0627395106303746,-0.0544016617342056,
-0.497967797283864));
#53967=CARTESIAN_POINT('Ctrl Pts',(0.079732977361713,0.0232047075568513,
-0.492411030241303));
#53968=CARTESIAN_POINT('Ctrl Pts',(0.0237488997309608,0.0795725784672084,
-0.486854263198742));
#53969=CARTESIAN_POINT('Ctrl Pts',(-0.0539718427219837,0.0631097514003656,
-0.481297496156181));
#53970=CARTESIAN_POINT('Ctrl Pts',(-0.0822936521765144,-0.0111156806028886,
-0.475740729113621));
#53971=CARTESIAN_POINT('Ctrl Pts',(-0.0352942967205491,-0.0751672522841446,
-0.470183962071058));
#53972=CARTESIAN_POINT('Ctrl Pts',(0.0440089628392656,-0.070420265167342,
-0.464627195028499));
#53973=CARTESIAN_POINT('Ctrl Pts',(0.0830320165918719,-0.00121952455203425,
-0.459070427985936));
#53974=CARTESIAN_POINT('Ctrl Pts',(0.0460581145487806,0.0690974168616255,
-0.453513660943376));
#53975=CARTESIAN_POINT('Ctrl Pts',(-0.0330715296041798,0.0761713645877082,
-0.447956893900814));
#53976=CARTESIAN_POINT('Ctrl Pts',(-0.0819317001146608,0.0135277285341473,
-0.442400126858254));
#53977=CARTESIAN_POINT('Ctrl Pts',(-0.0558020067273405,-0.061497471090078,
-0.436843359815692));
#53978=CARTESIAN_POINT('Ctrl Pts',(0.0214017501633328,-0.0802357026891362,
-0.431286592773131));
#53979=CARTESIAN_POINT('Ctrl Pts',(0.0790170655349912,-0.0255363713260351,
-0.42572982573057));
#53980=CARTESIAN_POINT('Ctrl Pts',(0.0643102033120854,0.052535708360603,
-0.420173058688009));
#53981=CARTESIAN_POINT('Ctrl Pts',(-0.00925804420869325,0.0825232786518928,
-0.414616291645448));
#53982=CARTESIAN_POINT('Ctrl Pts',(-0.0743526549108956,0.0369795296237106,
-0.409059524602887));
#53983=CARTESIAN_POINT('Ctrl Pts',(-0.0713942966320421,-0.0424105801815723,
-0.403502757560325));
#53984=CARTESIAN_POINT('Ctrl Pts',(-0.00309067450077944,-0.0829834359012095,
-0.397945990517765));
#53985=CARTESIAN_POINT('Ctrl Pts',(0.0680417581997704,-0.0476038028326378,
-0.392389223475203));
#53986=CARTESIAN_POINT('Ctrl Pts',(0.0768974145659965,0.0313463001966025,
-0.386832456432643));
#53987=CARTESIAN_POINT('Ctrl Pts',(0.0153709524480465,0.0816059846076698,
-0.381275689390081));
#53988=CARTESIAN_POINT('Ctrl Pts',(-0.0602241256637174,0.0571739240477337,
-0.37571892234752));
#53989=CARTESIAN_POINT('Ctrl Pts',(-0.0806976945278576,-0.0195878789267407,
-0.370162155304959));
#53990=CARTESIAN_POINT('Ctrl Pts',(-0.0273108517025254,-0.0784214274432931,
-0.364605388262398));
#53991=CARTESIAN_POINT('Ctrl Pts',(0.0510728731545283,-0.0654779698120381,
-0.359048621219837));
#53992=CARTESIAN_POINT('Ctrl Pts',(0.0827109820502502,0.00739569815808381,
-0.353491854177276));
#53993=CARTESIAN_POINT('Ctrl Pts',(0.0386459717773164,0.0735002841378828,
-0.347935087134715));
#53994=CARTESIAN_POINT('Ctrl Pts',(-0.0407906485808458,0.0723320530008452,
-0.342378320092154));
#53995=CARTESIAN_POINT('Ctrl Pts',(-0.0828926943282594,0.00496025503019042,
-0.336821553049593));
#53996=CARTESIAN_POINT('Ctrl Pts',(-0.0491253045860583,-0.066951529872661,
-0.331264786007031));
#53997=CARTESIAN_POINT('Ctrl Pts',(0.0296051444149024,-0.077584394868657,
-0.325708018964471));
#53998=CARTESIAN_POINT('Ctrl Pts',(0.0812388074741194,-0.0172063669362776,
-0.320151251921909));
#53999=CARTESIAN_POINT('Ctrl Pts',(0.0585167928362994,0.0589201821035582,
-0.314594484879348));
#54000=CARTESIAN_POINT('Ctrl Pts',(-0.0177640556062421,0.0811186860802194,
-0.309037717836787));
#54001=CARTESIAN_POINT('Ctrl Pts',(-0.0777859456233938,0.0290714562145981,
-0.303480950794226));
#54002=CARTESIAN_POINT('Ctrl Pts',(-0.0666124687713937,-0.0495840892539429,
-0.297924183751665));
#54003=CARTESIAN_POINT('Ctrl Pts',(0.00552959455508908,-0.0828566622971212,
-0.292367416709103));
#54004=CARTESIAN_POINT('Ctrl Pts',(0.0726105699198304,-0.0402927789917783,
-0.286810649666543));
#54005=CARTESIAN_POINT('Ctrl Pts',(0.0732330594669769,0.0391499923891321,
-0.281253882623981));
#54006=CARTESIAN_POINT('Ctrl Pts',(0.00682731539278151,0.0827598372853061,
-0.275697115581421));
#54007=CARTESIAN_POINT('Ctrl Pts',(-0.0658272853382939,0.0506218471408707,
-0.270140348538859));
#54008=CARTESIAN_POINT('Ctrl Pts',(-0.0782319567010151,-0.0278489470841068,
-0.264583581496299));
#54009=CARTESIAN_POINT('Ctrl Pts',(-0.0190330393487936,-0.0808303551650625,
-0.259026814453737));
#54010=CARTESIAN_POINT('Ctrl Pts',(0.0575863028399786,-0.0598299308723078,
-0.253470047411176));
#54011=CARTESIAN_POINT('Ctrl Pts',(0.0814984634874966,0.0159312068638903,
-0.247913280368615));
#54012=CARTESIAN_POINT('Ctrl Pts',(0.0308172903294861,0.07711094293102,
-0.242356513326054));
#54013=CARTESIAN_POINT('Ctrl Pts',(-0.0480701130586427,0.0677131237906815,
-0.236799746283493));
#54014=CARTESIAN_POINT('Ctrl Pts',(-0.0829602453816192,-0.00366068151911704,
-0.231242979240932));
#54015=CARTESIAN_POINT('Ctrl Pts',(-0.0419191145674805,-0.0716839642935664,
-0.225686212198371));
#54016=CARTESIAN_POINT('Ctrl Pts',(0.0374894451767004,-0.0740968582552996,
-0.22012944515581));
#54017=CARTESIAN_POINT('Ctrl Pts',(0.0825849322740763,-0.00869090698657777,
-0.214572678113249));
#54018=CARTESIAN_POINT('Ctrl Pts',(0.05209267014508,0.0646695957936844,
-0.209015911070688));
#54019=CARTESIAN_POINT('Ctrl Pts',(-0.0260786004789479,0.0788397710551074,
-0.203459144028126));
#54020=CARTESIAN_POINT('Ctrl Pts',(-0.0803808352038637,0.020850041604132,
-0.197902376985565));
#54021=CARTESIAN_POINT('Ctrl Pts',(-0.0611126709868174,-0.0562231655798389,
-0.192345609943004));
#54022=CARTESIAN_POINT('Ctrl Pts',(0.0140902639190115,-0.0818368337953801,
-0.186788842900443));
#54023=CARTESIAN_POINT('Ctrl Pts',(0.0763967623163283,-0.0325474670375087,
-0.181232075857882));
#54024=CARTESIAN_POINT('Ctrl Pts',(0.0687793756575961,0.0465317137777947,
-0.175675308815321));
#54025=CARTESIAN_POINT('Ctrl Pts',(-0.00178990859256147,0.0830216786759971,
-0.17011854177276));
#54026=CARTESIAN_POINT('Ctrl Pts',(-0.0707209380421003,0.0435241522087464,
-0.164561774730199));
#54027=CARTESIAN_POINT('Ctrl Pts',(-0.0749230104927655,-0.0358098506215939,
-0.159005007687638));
#54028=CARTESIAN_POINT('Ctrl Pts',(-0.010550082974379,-0.0823680681584513,
-0.153448240645076));
#54029=CARTESIAN_POINT('Ctrl Pts',(0.0634790494320266,-0.0535370263154007,
-0.147891473602516));
#54030=CARTESIAN_POINT('Ctrl Pts',(0.0794075291109813,0.0242950040649667,
-0.142334706559954));
#54031=CARTESIAN_POINT('Ctrl Pts',(0.0226564505462031,0.0798904759757979,
-0.136777939517394));
#54032=CARTESIAN_POINT('Ctrl Pts',(-0.0548314629182453,0.0623643614615536,
-0.131221172474832));
#54033=CARTESIAN_POINT('Ctrl Pts',(-0.0821336250436817,-0.0122421621152916,
-0.125664405432271));
#54034=CARTESIAN_POINT('Ctrl Pts',(-0.034261107366836,-0.0756437666121359,
-0.12010763838971));
#54035=CARTESIAN_POINT('Ctrl Pts',(0.0449696731861309,-0.0698106826818423,
-0.114550871347149));
#54036=CARTESIAN_POINT('Ctrl Pts',(0.0830409306702594,-8.1773656234945E-5,
-0.108994104304588));
#54037=CARTESIAN_POINT('Ctrl Pts',(0.0451070770045397,0.069721980299217,
-0.103437337262027));
#54038=CARTESIAN_POINT('Ctrl Pts',(-0.0341120631480026,0.0757110967245396,
-0.0978805702194658));
#54039=CARTESIAN_POINT('Ctrl Pts',(-0.0821093530945509,0.0124038982106829,
-0.0923238031769044));
#54040=CARTESIAN_POINT('Ctrl Pts',(-0.0549541856563936,-0.0622562500941794,
-0.0867670361343436));
#54041=CARTESIAN_POINT('Ctrl Pts',(0.0224990713206748,-0.079934944383053,
-0.0812102690917824));
#54042=CARTESIAN_POINT('Ctrl Pts',(0.0793595128123734,-0.0244513446420697,
-0.0756535020492213));
#54043=CARTESIAN_POINT('Ctrl Pts',(0.0635843925206498,0.0534118948374907,
-0.0700967350066603));
#54044=CARTESIAN_POINT('Ctrl Pts',(-0.0103878900392474,0.0823886999065706,
-0.064539967964099));
#54045=CARTESIAN_POINT('Ctrl Pts',(-0.0748522443330048,0.0359573151374515,
-0.0589832009215382));
#54046=CARTESIAN_POINT('Ctrl Pts',(-0.0708066992009198,-0.0433847365203528,
-0.0534264338789768));
#54047=CARTESIAN_POINT('Ctrl Pts',(-0.00195307623790311,-0.0830180833226157,
-0.0478696668364159));
#54048=CARTESIAN_POINT('Ctrl Pts',(0.0686869577732957,-0.0466669108006935,
-0.0423128997938547));
#54049=CARTESIAN_POINT('Ctrl Pts',(0.0764619314007254,0.0323966156580473,
-0.0367561327512937));
#54050=CARTESIAN_POINT('Ctrl Pts',(0.0142491077581508,0.0818095435552619,
-0.0311993657087326));
#54051=CARTESIAN_POINT('Ctrl Pts',(-0.0609974528606526,0.0563422431806374,
-0.0256425986661715));
#54052=CARTESIAN_POINT('Ctrl Pts',(-0.080430027617677,-0.0206894676307396,
-0.0200858316236103));
#54053=CARTESIAN_POINT('Ctrl Pts',(-0.0262181045220728,-0.0787924811616626,
-0.0145290645810493));
#54054=CARTESIAN_POINT('Ctrl Pts',(0.051935294733289,-0.0647640088968256,
-0.00897229753848818));
#54055=CARTESIAN_POINT('Ctrl Pts',(0.0826595173397112,0.00851255801366293,
-0.00341553049592713));
#54056=CARTESIAN_POINT('Ctrl Pts',(0.0375182880181104,0.0740559929469865,
0.00214123654663404));
#54057=CARTESIAN_POINT('Ctrl Pts',(-0.0151567811149895,0.0724726838097691,
0.00584574790834138));
#54058=CARTESIAN_POINT('Ctrl Pts',(-0.0353469172674506,0.0607192625322951,
0.00769800358919507));
#54059=CARTESIAN_POINT('Ctrl Pts',(0.0763850617480247,-0.00909823976109972,
-0.5608));
#54060=CARTESIAN_POINT('Ctrl Pts',(0.0794103735167017,0.0163010278253026,
-0.558947744319146));
#54061=CARTESIAN_POINT('Ctrl Pts',(0.0580845843294891,0.0699146924242753,
-0.555243232957439));
#54062=CARTESIAN_POINT('Ctrl Pts',(-0.0274085988114208,0.0867549003063301,
-0.549686465914878));
#54063=CARTESIAN_POINT('Ctrl Pts',(-0.0876658603765707,0.0240055824336086,
-0.544129698872316));
#54064=CARTESIAN_POINT('Ctrl Pts',(-0.0677597442009021,-0.0606215649972542,
-0.538572931829756));
#54065=CARTESIAN_POINT('Ctrl Pts',(0.0142039975012356,-0.0898124769136294,
-0.533016164787195));
#54066=CARTESIAN_POINT('Ctrl Pts',(0.0831467079379578,-0.0367746500978545,
-0.527459397744632));
#54067=CARTESIAN_POINT('Ctrl Pts',(0.0759982965549535,0.0499084064654446,
-0.521902630702073));
#54068=CARTESIAN_POINT('Ctrl Pts',(-0.000714994011805219,0.0909188305374142,
-0.51634586365951));
#54069=CARTESIAN_POINT('Ctrl Pts',(-0.076770863805945,0.0487099276131553,
-0.510789096616951));
#54070=CARTESIAN_POINT('Ctrl Pts',(-0.0825620293213013,-0.0380798538367916,
-0.505232329574389));
#54071=CARTESIAN_POINT('Ctrl Pts',(-0.0127855715928567,-0.0900172312567932,
-0.499675562531827));
#54072=CARTESIAN_POINT('Ctrl Pts',(0.0686927318976377,-0.0595637219153667,
-0.494118795489267));
#54073=CARTESIAN_POINT('Ctrl Pts',(0.0872986732328282,0.0254065538438251,
-0.488562028446705));
#54074=CARTESIAN_POINT('Ctrl Pts',(0.0260023832779629,0.0871230544218715,
-0.483005261404145));
#54075=CARTESIAN_POINT('Ctrl Pts',(-0.059093118273826,0.0690981040418431,
-0.477448494361583));
#54076=CARTESIAN_POINT('Ctrl Pts',(-0.0901023251383473,-0.012170424344118,
-0.471891727319023));
#54077=CARTESIAN_POINT('Ctrl Pts',(-0.0386432989001772,-0.0822997160283402,
-0.46633496027646));
#54078=CARTESIAN_POINT('Ctrl Pts',(0.0481848815050713,-0.077102297207892,
-0.460778193233902));
#54079=CARTESIAN_POINT('Ctrl Pts',(0.0909107514125927,-0.00133524269242489,
-0.455221426191338));
#54080=CARTESIAN_POINT('Ctrl Pts',(0.0504284729450598,0.0756539265863672,
-0.449664659148779));
#54081=CARTESIAN_POINT('Ctrl Pts',(-0.0362096180496001,0.0833991064534618,
-0.444107892106217));
#54082=CARTESIAN_POINT('Ctrl Pts',(-0.089706028200502,0.0148113464712039,
-0.438551125063656));
#54083=CARTESIAN_POINT('Ctrl Pts',(-0.0610969427232932,-0.0673328378166892,
-0.432994358021095));
#54084=CARTESIAN_POINT('Ctrl Pts',(0.0234325175848321,-0.0878491011177105,
-0.427437590978534));
#54085=CARTESIAN_POINT('Ctrl Pts',(0.0865148300265095,-0.027959464323406,
-0.421880823935973));
#54086=CARTESIAN_POINT('Ctrl Pts',(0.0704124643309056,0.0575207121191699,
-0.416324056893412));
#54087=CARTESIAN_POINT('Ctrl Pts',(-0.0101365207081535,0.0903537403908936,
-0.41076728985085));
#54088=CARTESIAN_POINT('Ctrl Pts',(-0.0814078232098771,0.0404884400375374,
-0.405210522808289));
#54089=CARTESIAN_POINT('Ctrl Pts',(-0.0781687524861088,-0.0464348316517719,
-0.399653755765728));
#54090=CARTESIAN_POINT('Ctrl Pts',(-0.00338394215593656,-0.0908575610015496,
-0.394096988723167));
#54091=CARTESIAN_POINT('Ctrl Pts',(0.07449809867656,-0.0521208283653285,
-0.388540221680606));
#54092=CARTESIAN_POINT('Ctrl Pts',(0.084194049799397,0.0343206852229668,
-0.382983454638044));
#54093=CARTESIAN_POINT('Ctrl Pts',(0.0168294700566864,0.0893494062286084,
-0.377426687595484));
#54094=CARTESIAN_POINT('Ctrl Pts',(-0.0659386672994629,0.0625990384159216,
-0.371869920552922));
#54095=CARTESIAN_POINT('Ctrl Pts',(-0.0883549303981324,-0.0214465318909665,
-0.366313153510362));
#54096=CARTESIAN_POINT('Ctrl Pts',(-0.0299023214406378,-0.0858626730789984,
-0.3607563864678));
#54097=CARTESIAN_POINT('Ctrl Pts',(0.055919071532374,-0.0716910377576715,
-0.35519961942524));
#54098=CARTESIAN_POINT('Ctrl Pts',(0.0905592545731065,0.00809746052630369,
-0.349642852382678));
#54099=CARTESIAN_POINT('Ctrl Pts',(0.0423130074103206,0.0804745727525552,
-0.344086085340117));
#54100=CARTESIAN_POINT('Ctrl Pts',(-0.0446611881211935,0.0791954906002617,
-0.338529318297556));
#54101=CARTESIAN_POINT('Ctrl Pts',(-0.0907582091500607,0.00543092328118761,
-0.332972551254996));
#54102=CARTESIAN_POINT('Ctrl Pts',(-0.053786702245749,-0.0733044208580867,
-0.327415784212434));
#54103=CARTESIAN_POINT('Ctrl Pts',(0.032414314801798,-0.084946216229697,
-0.321859017169873));
#54104=CARTESIAN_POINT('Ctrl Pts',(0.0889473884229148,-0.0188390431963924,
-0.316302250127312));
#54105=CARTESIAN_POINT('Ctrl Pts',(0.0640693292221425,0.0645109952553602,
-0.310745483084751));
#54106=CARTESIAN_POINT('Ctrl Pts',(-0.0194496497807158,0.088815868960563,
-0.30518871604219));
#54107=CARTESIAN_POINT('Ctrl Pts',(-0.0851668917150452,0.0318299860416274,
-0.299631948999629));
#54108=CARTESIAN_POINT('Ctrl Pts',(-0.0729331869563206,-0.0542890200335835,
-0.294075181957068));
#54109=CARTESIAN_POINT('Ctrl Pts',(0.00605428624576221,-0.0907187581146632,
-0.288518414914506));
#54110=CARTESIAN_POINT('Ctrl Pts',(0.0795004354086054,-0.0441160767255499,
-0.282961647871945));
#54111=CARTESIAN_POINT('Ctrl Pts',(0.0801819916901514,0.0428648534864279,
-0.277404880829384));
#54112=CARTESIAN_POINT('Ctrl Pts',(0.00747514510624739,0.0906127455794876,
-0.271848113786823));
#54113=CARTESIAN_POINT('Ctrl Pts',(-0.0720734991054189,0.0554252486012789,
-0.266291346744262));
#54114=CARTESIAN_POINT('Ctrl Pts',(-0.0856552238532882,-0.0304914755703219,
-0.2607345797017));
#54115=CARTESIAN_POINT('Ctrl Pts',(-0.0208390447430576,-0.0885001789264252,
-0.25517781265914));
#54116=CARTESIAN_POINT('Ctrl Pts',(0.0630505469713957,-0.0655070681867248,
-0.249621045616578));
#54117=CARTESIAN_POINT('Ctrl Pts',(0.0892316826536689,0.0174428858451625,
-0.244064278574018));
#54118=CARTESIAN_POINT('Ctrl Pts',(0.0337414787132595,0.0844278394254827,
-0.238507511531456));
#54119=CARTESIAN_POINT('Ctrl Pts',(-0.0526313857957924,0.0741382808340391,
-0.232950744488896));
#54120=CARTESIAN_POINT('Ctrl Pts',(-0.090832169981939,-0.00400803595100973,
-0.227393977446334));
#54121=CARTESIAN_POINT('Ctrl Pts',(-0.0458967318909284,-0.078485906107687,
-0.221837210403773));
#54122=CARTESIAN_POINT('Ctrl Pts',(0.0410467404134879,-0.0811277545433131,
-0.216280443361212));
#54123=CARTESIAN_POINT('Ctrl Pts',(0.0904212441966549,-0.00951556901827846,
-0.210723676318651));
#54124=CARTESIAN_POINT('Ctrl Pts',(0.0570356349317089,0.0708059588152648,
-0.20516690927609));
#54125=CARTESIAN_POINT('Ctrl Pts',(-0.0285531444693586,0.086320712443328,
-0.199610142233528));
#54126=CARTESIAN_POINT('Ctrl Pts',(-0.0880080049539633,0.0228284585515061,
-0.194053375190968));
#54127=CARTESIAN_POINT('Ctrl Pts',(-0.066911524834458,-0.0615580644606202,
-0.188496608148406));
#54128=CARTESIAN_POINT('Ctrl Pts',(0.0154272596650918,-0.0896021602141092,
-0.182939841105846));
#54129=CARTESIAN_POINT('Ctrl Pts',(0.0836458917022921,-0.0356358282793559,
-0.177383074063284));
#54130=CARTESIAN_POINT('Ctrl Pts',(0.0753057071160328,0.0509470110168211,
-0.171826307020724));
#54131=CARTESIAN_POINT('Ctrl Pts',(-0.00195974928453672,0.0908994325534489,
-0.166269539978162));
#54132=CARTESIAN_POINT('Ctrl Pts',(-0.0774315003044271,0.0476540682053071,
-0.160712772935601));
#54133=CARTESIAN_POINT('Ctrl Pts',(-0.0820322986429512,-0.0392077726352661,
-0.15515600589304));
#54134=CARTESIAN_POINT('Ctrl Pts',(-0.0115511583366739,-0.0901838022975522,
-0.149599238850479));
#54135=CARTESIAN_POINT('Ctrl Pts',(0.0695024439932433,-0.0586170430456018,
-0.144042471807918));
#54136=CARTESIAN_POINT('Ctrl Pts',(0.0869423438765829,0.0266003063128576,
-0.138485704765357));
#54137=CARTESIAN_POINT('Ctrl Pts',(0.0248062738692927,0.0874711165618063,
-0.132928937722796));
#54138=CARTESIAN_POINT('Ctrl Pts',(-0.060034306037044,0.06828198560688,
-0.127372170680234));
#54139=CARTESIAN_POINT('Ctrl Pts',(-0.0899271133647523,-0.0134037953370005,
-0.121815403637674));
#54140=CARTESIAN_POINT('Ctrl Pts',(-0.0375120723642829,-0.0828214458067399,
-0.116258636595112));
#54141=CARTESIAN_POINT('Ctrl Pts',(0.0492367516523744,-0.0764348727121444,
-0.110701869552552));
#54142=CARTESIAN_POINT('Ctrl Pts',(0.0909205113292806,-8.95329878673978E-5,
-0.10514510250999));
#54143=CARTESIAN_POINT('Ctrl Pts',(0.0493871934324411,0.0763377535454949,
-0.0995883354674292));
#54144=CARTESIAN_POINT('Ctrl Pts',(-0.0373488856504812,0.0828951647330362,
-0.0940315684248683));
#54145=CARTESIAN_POINT('Ctrl Pts',(-0.0899005383010079,0.013580878233047,
-0.0884748013823069));
#54146=CARTESIAN_POINT('Ctrl Pts',(-0.0601686736797739,-0.0681636157774126,
-0.0829180343397461));
#54147=CARTESIAN_POINT('Ctrl Pts',(0.0246339612574005,-0.0875198044834496,
-0.0773612672971848));
#54148=CARTESIAN_POINT('Ctrl Pts',(0.0868897714115783,-0.0267714817211423,
-0.0718045002546238));
#54149=CARTESIAN_POINT('Ctrl Pts',(0.0696177828677645,0.0584800381028195,
-0.0662477332120627));
#54150=CARTESIAN_POINT('Ctrl Pts',(-0.0113735752523172,0.0902063917492059,
-0.0606909661695015));
#54151=CARTESIAN_POINT('Ctrl Pts',(-0.0819548176299329,0.0393692297513722,
-0.0551341991269405));
#54152=CARTESIAN_POINT('Ctrl Pts',(-0.0775253991606801,-0.0475014236531102,
-0.0495774320843793));
#54153=CARTESIAN_POINT('Ctrl Pts',(-0.00213839956732174,-0.0908954960444865,
-0.0440206650418183));
#54154=CARTESIAN_POINT('Ctrl Pts',(0.0752045198915063,-0.0510950366031558,
-0.0384638979992572));
#54155=CARTESIAN_POINT('Ctrl Pts',(0.0837172445451427,0.0354706629272246,
-0.0329071309566961));
#54156=CARTESIAN_POINT('Ctrl Pts',(0.0156011758647249,0.0895722804600428,
-0.0273503639141351));
#54157=CARTESIAN_POINT('Ctrl Pts',(-0.0667853739006856,0.0616884410865223,
-0.0217935968715739));
#54158=CARTESIAN_POINT('Ctrl Pts',(-0.0880618651332911,-0.0226526480487904,
-0.0162368298290128));
#54159=CARTESIAN_POINT('Ctrl Pts',(-0.0287058857600831,-0.0862689353105569,
-0.0106800627864517));
#54160=CARTESIAN_POINT('Ctrl Pts',(0.0568633264954318,-0.0709093305807852,
-0.00512329574389066));
#54161=CARTESIAN_POINT('Ctrl Pts',(0.0905029064835577,0.00932029688342027,
0.000433471298670411));
#54162=CARTESIAN_POINT('Ctrl Pts',(0.0410783200919443,0.0810830116111529,
0.00599023834123158));
#54163=CARTESIAN_POINT('Ctrl Pts',(-0.0165949764526702,0.0793494655732392,
0.00969474970293892));
#54164=CARTESIAN_POINT('Ctrl Pts',(-0.0387009125009883,0.0664807866724729,
0.0115470053837926));
#54165=CARTESIAN_POINT('',(0.0769008389612107,0.00192784648297797,0.));
#54166=CARTESIAN_POINT('Ctrl Pts',(0.0770242870977014,0.00196088950922314,
-1.56125112837913E-17));
#54167=CARTESIAN_POINT('Ctrl Pts',(0.0767355444305697,0.00393482941033669,
-2.03122860241009E-17));
#54168=CARTESIAN_POINT('Ctrl Pts',(0.0763650804585085,0.00589328886515121,
4.04310519118361E-17));
#54169=CARTESIAN_POINT('Ctrl Pts',(0.0759106818058855,0.00783195085873916,
3.12250225675825E-17));
#54170=CARTESIAN_POINT('Ctrl Pts',(0.0749514899506794,0.011924279881973,
1.18503374704373E-17));
#54171=CARTESIAN_POINT('Ctrl Pts',(0.0736187376959688,0.0159288611658458,
-4.04200893462907E-17));
#54172=CARTESIAN_POINT('Ctrl Pts',(0.0719425060131334,0.0198063602908007,
-8.67361737988404E-18));
#54173=CARTESIAN_POINT('Ctrl Pts',(0.070871047943992,0.0222848826621795,
1.16189316176618E-17));
#54174=CARTESIAN_POINT('Ctrl Pts',(0.0696591442633312,0.0247101164831124,
2.15812243806632E-17));
#54175=CARTESIAN_POINT('Ctrl Pts',(0.0683207983996043,0.0270604039630841,
1.90819582357449E-17));
#54176=CARTESIAN_POINT('Ctrl Pts',(0.0667211506419413,0.0298695672736282,
1.60947293042127E-17));
#54177=CARTESIAN_POINT('Ctrl Pts',(0.0649390499018336,0.032576338574731,
-1.48038691071277E-16));
#54178=CARTESIAN_POINT('Ctrl Pts',(0.06298781283264,0.0351614966284854,
-1.6306400674182E-16));
#54179=CARTESIAN_POINT('Ctrl Pts',(0.0610180171756984,0.0377712426133224,
-1.78232231054124E-16));
#54180=CARTESIAN_POINT('Ctrl Pts',(0.0588721823446311,0.0402598580152677,
-6.31405163010684E-17));
#54181=CARTESIAN_POINT('Ctrl Pts',(0.0565835086679188,0.0425851086778113,
-3.46944695195361E-17));
#54182=CARTESIAN_POINT('Ctrl Pts',(0.0526077988759246,0.0466243572268643,
1.47198388126686E-17));
#54183=CARTESIAN_POINT('Ctrl Pts',(0.0481933888539555,0.0501870891976839,
-4.56922916309108E-18));
#54184=CARTESIAN_POINT('Ctrl Pts',(0.0434112988581259,0.0531552124976776,
5.20417042793042E-18));
#54185=CARTESIAN_POINT('Ctrl Pts',(0.0406871449609811,0.054846026485272,
1.07716617565028E-17));
#54186=CARTESIAN_POINT('Ctrl Pts',(0.0378378243539425,0.0563447142077944,
-1.15248730856744E-16));
#54187=CARTESIAN_POINT('Ctrl Pts',(0.0349064264744822,0.0576115805932702,
-8.15320033709099E-17));
#54188=CARTESIAN_POINT('Ctrl Pts',(0.0333579064157681,0.0582808067066427,
-6.37210370766907E-17));
#54189=CARTESIAN_POINT('Ctrl Pts',(0.0317852908376245,0.0588862744051351,
-6.38585590855274E-17));
#54190=CARTESIAN_POINT('Ctrl Pts',(0.0301905740463167,0.0594245974561285,
-6.33174068731535E-17));
#54191=CARTESIAN_POINT('Ctrl Pts',(0.0271332970740427,0.0604566319066448,
-6.31473102947789E-17));
#54192=CARTESIAN_POINT('Ctrl Pts',(0.0239946807002247,0.0612421909225445,
1.57144674071977E-16));
#54193=CARTESIAN_POINT('Ctrl Pts',(0.0208030260208049,0.0617831377165539,
1.62196645003831E-16));
#54194=CARTESIAN_POINT('Ctrl Pts',(0.0186151991120485,0.0621539478670914,
1.65659688176464E-16));
#54195=CARTESIAN_POINT('Ctrl Pts',(0.0164005708805104,0.062409806097221,
-6.83477658214862E-17));
#54196=CARTESIAN_POINT('Ctrl Pts',(0.0141748740344104,0.0625496135305,-5.8113236445223E-17));
#54197=CARTESIAN_POINT('Ctrl Pts',(0.00874673157748686,0.0628905829961777,
-3.31527466411991E-17));
#54198=CARTESIAN_POINT('Ctrl Pts',(0.00329440124118755,0.0625432479469995,
1.08495009030099E-16));
#54199=CARTESIAN_POINT('Ctrl Pts',(-0.0020407491023474,0.0615174160184291,
1.04950770296597E-16));
#54200=CARTESIAN_POINT('Ctrl Pts',(-0.0041885001110211,0.061104450793937,
1.0352397970501E-16));
#54201=CARTESIAN_POINT('Ctrl Pts',(-0.00631700386563472,0.0605810109679865,
-2.68752568833808E-17));
#54202=CARTESIAN_POINT('Ctrl Pts',(-0.0084154806475312,0.0599458611255486,
-3.07913416985883E-17));
#54203=CARTESIAN_POINT('Ctrl Pts',(-0.0105364069326447,0.0593039164505187,
-3.47493207865443E-17));
#54204=CARTESIAN_POINT('Ctrl Pts',(-0.0126184161606321,0.0585501961183772,
-1.85078928243005E-17));
#54205=CARTESIAN_POINT('Ctrl Pts',(-0.0146468443017921,0.0576869532301707,
-2.64545330086463E-17));
#54206=CARTESIAN_POINT('Ctrl Pts',(-0.0192232633510667,0.0557393559169726,
-4.43832704282387E-17));
#54207=CARTESIAN_POINT('Ctrl Pts',(-0.0235379545271893,0.0532336481116517,
-3.79989797786901E-17));
#54208=CARTESIAN_POINT('Ctrl Pts',(-0.0274528972419724,0.0501564562137779,
-2.07624716030974E-17));
#54209=CARTESIAN_POINT('Ctrl Pts',(-0.027852503585005,0.0498423608385185,
-1.90031053746486E-17));
#54210=CARTESIAN_POINT('Ctrl Pts',(-0.028247905322877,0.0495222895177995,
-1.23650236939171E-18));
#54211=CARTESIAN_POINT('Ctrl Pts',(-0.0286389268003753,0.0491962142519396,
0.));
#54212=CARTESIAN_POINT('Ctrl Pts',(-0.0769126606442387,-6.94072219677582E-5,
-0.0176396170927523));
#54213=CARTESIAN_POINT('Ctrl Pts',(-0.076971024511457,-0.0065279364822696,
-0.0171720213381724));
#54214=CARTESIAN_POINT('Ctrl Pts',(-0.0762252932793503,-0.0129732902276908,
-0.0167044255835926));
#54215=CARTESIAN_POINT('Ctrl Pts',(-0.074623120032322,-0.0191985144031997,
-0.0162368298290128));
#54216=CARTESIAN_POINT('Ctrl Pts',(-0.0682765386755549,-0.043858077136046,
-0.0143845741481591));
#54217=CARTESIAN_POINT('Ctrl Pts',(-0.0484912122178188,-0.0650635062233016,
-0.0125323184673054));
#54218=CARTESIAN_POINT('Ctrl Pts',(-0.0243370136130319,-0.0731062866453006,
-0.0106800627864517));
#54219=CARTESIAN_POINT('Ctrl Pts',(-0.000182815008244568,-0.0811490670672997,
-0.00882780710559804));
#54220=CARTESIAN_POINT('Ctrl Pts',(0.0283402557435934,-0.0760291988240425,
-0.00697555142474438));
#54221=CARTESIAN_POINT('Ctrl Pts',(0.0482083877842003,-0.0600976601250463,
-0.00512329574389069));
#54222=CARTESIAN_POINT('Ctrl Pts',(0.0665266501016693,-0.0454089060734496,
-0.00341553049592711));
#54223=CARTESIAN_POINT('Ctrl Pts',(0.0774876123484423,-0.0215294799140155,
-0.00170776524796349));
#54224=CARTESIAN_POINT('Ctrl Pts',(0.0770242870977013,0.00196088950922531,
1.00613961606655E-16));
#54225=CARTESIAN_POINT('',(-0.0213030042343889,0.0527886127454549,-0.5608));
#54226=CARTESIAN_POINT('Ctrl Pts',(-0.0213168644878943,0.0528821598543764,
-0.5608));
#54227=CARTESIAN_POINT('Ctrl Pts',(-0.0200400288559082,0.0536782786774046,
-0.5608));
#54228=CARTESIAN_POINT('Ctrl Pts',(-0.0187323017072707,0.0544185816222459,
-0.5608));
#54229=CARTESIAN_POINT('Ctrl Pts',(-0.0173965430020956,0.0551003306193025,
-0.5608));
#54230=CARTESIAN_POINT('Ctrl Pts',(-0.0144915803430684,0.0565829751804841,
-0.5608));
#54231=CARTESIAN_POINT('Ctrl Pts',(-0.0114545109907711,0.0577892023762642,
-0.5608));
#54232=CARTESIAN_POINT('Ctrl Pts',(-0.00832330515556293,0.0587308479779915,
-0.5608));
#54233=CARTESIAN_POINT('Ctrl Pts',(-0.00621786685346983,0.059364015141447,
-0.5608));
#54234=CARTESIAN_POINT('Ctrl Pts',(-0.00407091670421551,0.0598766588631911,
-0.5608));
#54235=CARTESIAN_POINT('Ctrl Pts',(-0.00190319110591001,0.0602702142526908,
-0.5608));
#54236=CARTESIAN_POINT('Ctrl Pts',(0.00195266903242079,0.060970254211523,
-0.5608));
#54237=CARTESIAN_POINT('Ctrl Pts',(0.00588166571401474,0.061296842042279,
-0.5608));
#54238=CARTESIAN_POINT('Ctrl Pts',(0.00982578190433832,0.0612640784166091,
-0.5608));
#54239=CARTESIAN_POINT('Ctrl Pts',(0.0120694902474667,0.0612454400153249,
-0.5608));
#54240=CARTESIAN_POINT('Ctrl Pts',(0.0143086737138421,0.0611103104399024,
-0.5608));
#54241=CARTESIAN_POINT('Ctrl Pts',(0.0165324227803292,0.0608624325775255,
-0.5608));
#54242=CARTESIAN_POINT('Ctrl Pts',(0.020213063703421,0.0604521572375861,
-0.5608));
#54243=CARTESIAN_POINT('Ctrl Pts',(0.023851531624229,0.0597335279680504,
-0.5608));
#54244=CARTESIAN_POINT('Ctrl Pts',(0.027403304404835,0.0587159243115919,
-0.5608));
#54245=CARTESIAN_POINT('Ctrl Pts',(0.029552326701873,0.0581002168656603,
-0.5608));
#54246=CARTESIAN_POINT('Ctrl Pts',(0.0316696966121409,0.0573748722106627,
-0.5608));
#54247=CARTESIAN_POINT('Ctrl Pts',(0.0337457330178675,0.0565401986057516,
-0.5608));
#54248=CARTESIAN_POINT('Ctrl Pts',(0.0357573291778275,0.0557314332999855,
-0.5608));
#54249=CARTESIAN_POINT('Ctrl Pts',(0.0377218002147095,0.0548232331313804,
-0.5608));
#54250=CARTESIAN_POINT('Ctrl Pts',(0.0396284595471832,0.0538189834925058,
-0.5608));
#54251=CARTESIAN_POINT('Ctrl Pts',(0.0407788604385921,0.0532130600010453,
-0.5608));
#54252=CARTESIAN_POINT('Ctrl Pts',(0.0419084909952876,0.0525720444311966,
-0.5608));
#54253=CARTESIAN_POINT('Ctrl Pts',(0.0430155335449313,0.0518963074449715,
-0.5608));
#54254=CARTESIAN_POINT('Ctrl Pts',(0.0469905641944571,0.0494699551497256,
-0.5608));
#54255=CARTESIAN_POINT('Ctrl Pts',(0.0506750453636331,0.0465978050955386,
-0.5608));
#54256=CARTESIAN_POINT('Ctrl Pts',(0.0540463165810115,0.0433542137292111,
-0.5608));
#54257=CARTESIAN_POINT('Ctrl Pts',(0.05564618250959,0.0418149393787913,
-0.5608));
#54258=CARTESIAN_POINT('Ctrl Pts',(0.0571743672102615,0.0401920536871288,
-0.5608));
#54259=CARTESIAN_POINT('Ctrl Pts',(0.0586198127704844,0.0385033456845963,
-0.5608));
#54260=CARTESIAN_POINT('Ctrl Pts',(0.0616266630685766,0.0349904550572784,
-0.5608));
#54261=CARTESIAN_POINT('Ctrl Pts',(0.0642868952611629,0.0311838839229392,
-0.5608));
#54262=CARTESIAN_POINT('Ctrl Pts',(0.0665797585803528,0.027151816035101,
-0.5608));
#54263=CARTESIAN_POINT('Ctrl Pts',(0.0678796009979006,0.0248660047409082,
-0.5608));
#54264=CARTESIAN_POINT('Ctrl Pts',(0.0690612345731456,0.0225073874127262,
-0.5608));
#54265=CARTESIAN_POINT('Ctrl Pts',(0.0701192745487128,0.0200863361487867,
-0.5608));
#54266=CARTESIAN_POINT('Ctrl Pts',(0.071030260471914,0.0180017801095736,
-0.5608));
#54267=CARTESIAN_POINT('Ctrl Pts',(0.0718473902749254,0.0158753395167728,
-0.5608));
#54268=CARTESIAN_POINT('Ctrl Pts',(0.0725655572330888,0.0137219177577617,
-0.5608));
#54269=CARTESIAN_POINT('Ctrl Pts',(0.0745600844141832,0.00774133318493183,
-0.5608));
#54270=CARTESIAN_POINT('Ctrl Pts',(0.0758018690746804,0.00153804309463624,
-0.5608));
#54271=CARTESIAN_POINT('Ctrl Pts',(0.0762248566852573,-0.00474661219965071,
-0.5608));
#54272=CARTESIAN_POINT('Ctrl Pts',(0.0763222229870443,-0.00619325893045234,
-0.5608));
#54273=CARTESIAN_POINT('Ctrl Pts',(0.0763760168749407,-0.00764432619612087,
-0.5608));
#54274=CARTESIAN_POINT('Ctrl Pts',(0.0763850617480247,-0.00909823976109944,
-0.5608));
#54275=CARTESIAN_POINT('Ctrl Pts',(-0.0213168644878947,0.0528821598543762,
-0.5608));
#54276=CARTESIAN_POINT('Ctrl Pts',(-0.0374049180327334,0.0462896122782152,
-0.559092234752037));
#54277=CARTESIAN_POINT('Ctrl Pts',(-0.0541768854252427,0.02761762516725,
-0.556887775577551));
#54278=CARTESIAN_POINT('Ctrl Pts',(-0.0569445161760761,0.00512363730287358,
-0.554683316403066));
#54279=CARTESIAN_POINT('Ctrl Pts',(-0.0569002140125902,4.52833130624442E-5,
-0.554186622476545));
#54280=CARTESIAN_POINT('Origin',(-8.56069748352724E-18,0.,-0.5608));
#54281=CARTESIAN_POINT('Ctrl Pts',(0.0402076065502267,-0.0657262044767394,
-0.5608));
#54282=CARTESIAN_POINT('Ctrl Pts',(0.0383936167831799,-0.066556416417856,
-0.5608));
#54283=CARTESIAN_POINT('Ctrl Pts',(0.0365482166471986,-0.0673096127760332,
-0.5608));
#54284=CARTESIAN_POINT('Ctrl Pts',(0.0346738275063863,-0.0679815896617125,
-0.5608));
#54285=CARTESIAN_POINT('Ctrl Pts',(0.0307171719732606,-0.0694000683569653,
-0.5608));
#54286=CARTESIAN_POINT('Ctrl Pts',(0.0266311929689044,-0.0704572681754979,
-0.5608));
#54287=CARTESIAN_POINT('Ctrl Pts',(0.0224652565211834,-0.0711570679346724,
-0.5608));
#54288=CARTESIAN_POINT('Ctrl Pts',(0.0198023631532829,-0.0716043844410448,
-0.5608));
#54289=CARTESIAN_POINT('Ctrl Pts',(0.0171078889170027,-0.0719048428903344,
-0.5608));
#54290=CARTESIAN_POINT('Ctrl Pts',(0.0144076243887813,-0.0720584304502345,
-0.5608));
#54291=CARTESIAN_POINT('Ctrl Pts',(0.0111801511265865,-0.0722420049622138,
-0.5608));
#54292=CARTESIAN_POINT('Ctrl Pts',(0.00793949242691801,-0.0722167745237351,
-0.5608));
#54293=CARTESIAN_POINT('Ctrl Pts',(0.00470902027438889,-0.0719834737466585,
-0.5608));
#54294=CARTESIAN_POINT('Ctrl Pts',(0.0014478283809384,-0.0717479544271862,
-0.5608));
#54295=CARTESIAN_POINT('Ctrl Pts',(-0.00180733306330198,-0.0712988329734778,
-0.5608));
#54296=CARTESIAN_POINT('Ctrl Pts',(-0.00500296882198629,-0.0706410311799038,
-0.5608));
#54297=CARTESIAN_POINT('Ctrl Pts',(-0.0105541900807911,-0.0694983467263818,
-0.5608));
#54298=CARTESIAN_POINT('Ctrl Pts',(-0.0159437658000986,-0.0677284487236317,
-0.5608));
#54299=CARTESIAN_POINT('Ctrl Pts',(-0.0210339685484103,-0.0653267882248462,
-0.5608));
#54300=CARTESIAN_POINT('Ctrl Pts',(-0.0239336398211533,-0.0639586647335923,
-0.5608));
#54301=CARTESIAN_POINT('Ctrl Pts',(-0.0267400378694071,-0.0623810675864798,
-0.5608));
#54302=CARTESIAN_POINT('Ctrl Pts',(-0.0293964253216744,-0.0606086000260937,
-0.5608));
#54303=CARTESIAN_POINT('Ctrl Pts',(-0.0307996708239191,-0.0596722881451354,
-0.5608));
#54304=CARTESIAN_POINT('Ctrl Pts',(-0.0321624853084298,-0.0586811031556425,
-0.5608));
#54305=CARTESIAN_POINT('Ctrl Pts',(-0.033480942421694,-0.0576348792224091,
-0.5608));
#54306=CARTESIAN_POINT('Ctrl Pts',(-0.0360085918225298,-0.0556291353333036,
-0.5608));
#54307=CARTESIAN_POINT('Ctrl Pts',(-0.0383735280098577,-0.0534211778677626,
-0.5608));
#54308=CARTESIAN_POINT('Ctrl Pts',(-0.040561936721919,-0.0510357775345927,
-0.5608));
#54309=CARTESIAN_POINT('Ctrl Pts',(-0.0420620578929242,-0.0494006215779431,
-0.5608));
#54310=CARTESIAN_POINT('Ctrl Pts',(-0.0434802420446818,-0.0476805031262554,
-0.5608));
#54311=CARTESIAN_POINT('Ctrl Pts',(-0.0448070177436098,-0.0458880324564179,
-0.5608));
#54312=CARTESIAN_POINT('Ctrl Pts',(-0.0480428217484688,-0.0415164692926221,
-0.5608));
#54313=CARTESIAN_POINT('Ctrl Pts',(-0.0507139486815803,-0.0367505873557775,
-0.5608));
#54314=CARTESIAN_POINT('Ctrl Pts',(-0.0527518145139489,-0.0317143920503034,
-0.5608));
#54315=CARTESIAN_POINT('Ctrl Pts',(-0.0535721880095819,-0.0296869959961479,
-0.5608));
#54316=CARTESIAN_POINT('Ctrl Pts',(-0.0542893617667917,-0.0276157278638674,
-0.5608));
#54317=CARTESIAN_POINT('Ctrl Pts',(-0.0548964411856249,-0.0255089656800579,
-0.5608));
#54318=CARTESIAN_POINT('Ctrl Pts',(-0.0555100186045104,-0.0233796533317132,
-0.5608));
#54319=CARTESIAN_POINT('Ctrl Pts',(-0.0560086146086451,-0.0212222738601327,
-0.5608));
#54320=CARTESIAN_POINT('Ctrl Pts',(-0.0563861523156285,-0.0190503620714463,
-0.5608));
#54321=CARTESIAN_POINT('Ctrl Pts',(-0.0572379279437924,-0.0141502382059215,
-0.5608));
#54322=CARTESIAN_POINT('Ctrl Pts',(-0.0574789598668102,-0.00916656265595418,
-0.5608));
#54323=CARTESIAN_POINT('Ctrl Pts',(-0.0570230227323766,-0.00420793446946095,
-0.5608));
#54324=CARTESIAN_POINT('Ctrl Pts',(-0.0569764839929469,-0.00370179384683607,
-0.5608));
#54325=CARTESIAN_POINT('Ctrl Pts',(-0.0569226437332971,-0.00319593569578702,
-0.5608));
#54326=CARTESIAN_POINT('Ctrl Pts',(-0.0568613829974075,-0.00269049226390578,
-0.5608));
#54327=CARTESIAN_POINT('Origin',(0.,0.,-0.5608));
#54328=CARTESIAN_POINT('Origin',(0.,0.,-0.648563377523455));
#54329=CARTESIAN_POINT('Ctrl Pts',(-0.0768390318326848,-0.00363576842162011,
-0.572347005383793));
#54330=CARTESIAN_POINT('Ctrl Pts',(-0.0756300800702637,-0.0291859883983543,
-0.570494749702939));
#54331=CARTESIAN_POINT('Ctrl Pts',(-0.0457466014776253,-0.0785438038026859,
-0.566790238341232));
#54332=CARTESIAN_POINT('Ctrl Pts',(0.0413535491490546,-0.0810402774590353,
-0.56123347129867));
#54333=CARTESIAN_POINT('Ctrl Pts',(0.0904258996703788,-0.00920489789578024,
-0.55567670425611));
#54334=CARTESIAN_POINT('Ctrl Pts',(0.0568231075837852,0.070975286479318,
-0.550119937213548));
#54335=CARTESIAN_POINT('Ctrl Pts',(-0.0288348405916419,0.0862356444712252,
-0.544563170170988));
#54336=CARTESIAN_POINT('Ctrl Pts',(-0.0880765772585221,0.0225447831988859,
-0.539006403128426));
#54337=CARTESIAN_POINT('Ctrl Pts',(-0.0667171067556589,-0.0617690697919249,
-0.533449636085865));
#54338=CARTESIAN_POINT('Ctrl Pts',(0.0157135236534292,-0.0895535055615975,
-0.527892869043304));
#54339=CARTESIAN_POINT('Ctrl Pts',(0.0837584047019811,-0.0353688086955708,
-0.522336102000743));
#54340=CARTESIAN_POINT('Ctrl Pts',(0.0751433811500897,0.0511862922340276,
-0.516779334958182));
#54341=CARTESIAN_POINT('Ctrl Pts',(-0.00224933968455702,0.0908928684440432,
-0.511222567915621));
#54342=CARTESIAN_POINT('Ctrl Pts',(-0.0775827744759656,0.0474071916605113,
-0.50566580087306));
#54343=CARTESIAN_POINT('Ctrl Pts',(-0.0819070771081818,-0.039468751630768,
-0.500109033830498));
#54344=CARTESIAN_POINT('Ctrl Pts',(-0.0112639065077944,-0.0902201489166854,
-0.494552266787938));
#54345=CARTESIAN_POINT('Ctrl Pts',(0.0696887350471192,-0.0583954204966491,
-0.488995499745376));
#54346=CARTESIAN_POINT('Ctrl Pts',(0.0868572077657704,0.0268770161445482,
-0.483438732702816));
#54347=CARTESIAN_POINT('Ctrl Pts',(0.0245276118500181,0.087549668072802,
-0.477881965660254));
#54348=CARTESIAN_POINT('Ctrl Pts',(-0.060251430791017,0.0680904724858967,
-0.472325198617693));
#54349=CARTESIAN_POINT('Ctrl Pts',(-0.0898839785216628,-0.0136900809031243,
-0.466768431575132));
#54350=CARTESIAN_POINT('Ctrl Pts',(-0.0372481547545244,-0.0829404772933564,
-0.461211664532571));
#54351=CARTESIAN_POINT('Ctrl Pts',(0.0494798934149131,-0.076277702240305,
-0.455654897490009));
#54352=CARTESIAN_POINT('Ctrl Pts',(0.0909203376627111,0.000199984617355618,
-0.450098130447449));
#54353=CARTESIAN_POINT('Ctrl Pts',(0.049143861682941,0.0764946313950189,
-0.444541363404887));
#54354=CARTESIAN_POINT('Ctrl Pts',(-0.0376126581190482,0.0827758159825542,
-0.438984596362327));
#54355=CARTESIAN_POINT('Ctrl Pts',(-0.0899433319377845,0.0132945407773614,
-0.433427829319765));
#54356=CARTESIAN_POINT('Ctrl Pts',(-0.0599513127724785,-0.0683548671821957,
-0.427871062277205));
#54357=CARTESIAN_POINT('Ctrl Pts',(0.0249125173624084,-0.0874409186145301,
-0.422314295234643));
#54358=CARTESIAN_POINT('Ctrl Pts',(0.0869745958753753,-0.0264946682098307,
-0.416757528192082));
#54359=CARTESIAN_POINT('Ctrl Pts',(0.0694311850831299,0.0587014336154286,
-0.411200761149521));
#54360=CARTESIAN_POINT('Ctrl Pts',(-0.0116607067891965,0.090169704932605,
-0.40564399410696));
#54361=CARTESIAN_POINT('Ctrl Pts',(-0.0820798699193133,0.0391080902720935,
-0.400087227064399));
#54362=CARTESIAN_POINT('Ctrl Pts',(-0.077373553700188,-0.0477480990029214,
-0.394530460021838));
#54363=CARTESIAN_POINT('Ctrl Pts',(-0.00184932175801734,-0.0909017479459029,
-0.388973692979277));
#54364=CARTESIAN_POINT('Ctrl Pts',(0.0753675442454562,-0.0508554917882798,
-0.383416925936715));
#54365=CARTESIAN_POINT('Ctrl Pts',(0.0836025405860219,0.0357374170605961,
-0.377860158894155));
#54366=CARTESIAN_POINT('Ctrl Pts',(0.0153183984047813,0.0896208370911247,
-0.372303391851593));
#54367=CARTESIAN_POINT('Ctrl Pts',(-0.0669862584792194,0.0614767349943143,
-0.366746624809033));
#54368=CARTESIAN_POINT('Ctrl Pts',(-0.0879802093044121,-0.0229353557058732,
-0.361189857766471));
#54369=CARTESIAN_POINT('Ctrl Pts',(-0.0284482601299106,-0.0863553372188681,
-0.35563309072391));
#54370=CARTESIAN_POINT('Ctrl Pts',(0.0571216101691189,-0.0707366200937766,
-0.350076323681349));
#54371=CARTESIAN_POINT('Ctrl Pts',(0.0904096195284211,0.00962540738513244,
-0.344519556638788));
#54372=CARTESIAN_POINT('Ctrl Pts',(0.0409481555832509,0.0811775604766097,
-0.338962789596227));
#54373=CARTESIAN_POINT('Ctrl Pts',(-0.045992044861177,0.0784300935871637,
-0.333406022553666));
#54374=CARTESIAN_POINT('Ctrl Pts',(-0.0908369737149324,0.00389768866334984,
-0.327849255511104));
#54375=CARTESIAN_POINT('Ctrl Pts',(-0.0525412835649756,-0.0742021650084995,
-0.322292488468544));
#54376=CARTESIAN_POINT('Ctrl Pts',(0.0338440187791357,-0.0843867890340737,
-0.316735721425982));
#54377=CARTESIAN_POINT('Ctrl Pts',(0.0892528084126734,-0.0173344731980629,
-0.311178954383422));
#54378=CARTESIAN_POINT('Ctrl Pts',(0.0629709225891355,0.0655836159332256,
-0.30562218734086));
#54379=CARTESIAN_POINT('Ctrl Pts',(-0.020946541228509,0.0884747996955411,
-0.300065420298299));
#54380=CARTESIAN_POINT('Ctrl Pts',(-0.0856922038235555,0.0303873982839258,
-0.294508653255739));
#54381=CARTESIAN_POINT('Ctrl Pts',(-0.0720061157964265,-0.0555127648249965,
-0.288951886213176));
#54382=CARTESIAN_POINT('Ctrl Pts',(0.00758521757887318,-0.0906035995139536,
-0.283395119170616));
#54383=CARTESIAN_POINT('Ctrl Pts',(0.080234006976822,-0.0427674162774302,
-0.277838352128054));
#54384=CARTESIAN_POINT('Ctrl Pts',(0.0794467853278221,0.0442126234426178,
-0.272281585085494));
#54385=CARTESIAN_POINT('Ctrl Pts',(0.00594407526174785,0.0907260477475264,
-0.266724818042932));
#54386=CARTESIAN_POINT('Ctrl Pts',(-0.0729990857182597,0.0542003805789396,
-0.261168051000372));
#54387=CARTESIAN_POINT('Ctrl Pts',(-0.0851281629049463,-0.031933425294394,
-0.25561128395781));
#54388=CARTESIAN_POINT('Ctrl Pts',(-0.019341740828334,-0.0888394328681432,
-0.250054516915249));
#54389=CARTESIAN_POINT('Ctrl Pts',(0.0641476521786357,-0.064433116412079,
-0.244497749872688));
#54390=CARTESIAN_POINT('Ctrl Pts',(0.0889244385051616,0.0189470843969588,
-0.238940982830127));
#54391=CARTESIAN_POINT('Ctrl Pts',(0.0323110974472321,0.0849855326061983,
-0.233384215787566));
#54392=CARTESIAN_POINT('Ctrl Pts',(-0.0538757149912223,0.0732390271971729,
-0.227827448745005));
#54393=CARTESIAN_POINT('Ctrl Pts',(-0.0907515463340875,-0.00554117393482795,
-0.222270681702444));
#54394=CARTESIAN_POINT('Ctrl Pts',(-0.0445649480385644,-0.0792496888127868,
-0.216713914659883));
#54395=CARTESIAN_POINT('Ctrl Pts',(0.0424107388215024,-0.0804231123696258,
-0.211157147617321));
#54396=CARTESIAN_POINT('Ctrl Pts',(0.0905690264021953,-0.0079874418410624,
-0.20560038057476));
#54397=CARTESIAN_POINT('Ctrl Pts',(0.0558319398891111,0.0717589176257572,
-0.200043613532199));
#54398=CARTESIAN_POINT('Ctrl Pts',(-0.0300066073256354,0.0858262855272531,
-0.194486846489638));
#54399=CARTESIAN_POINT('Ctrl Pts',(-0.088380920482232,0.0213391814588081,
-0.188930079447077));
#54400=CARTESIAN_POINT('Ctrl Pts',(-0.0658625735630241,-0.0626790967886454,
-0.183373312404516));
#54401=CARTESIAN_POINT('Ctrl Pts',(0.0169380010792513,-0.089328897284294,
-0.177816545361955));
#54402=CARTESIAN_POINT('Ctrl Pts',(0.0842356826073205,-0.0342183802419164,
-0.172259778319394));
#54403=CARTESIAN_POINT('Ctrl Pts',(0.0744347278870117,0.052211292407325,
-0.166703011276833));
#54404=CARTESIAN_POINT('Ctrl Pts',(-0.00349431497263191,0.0908533848209656,
-0.161146244234271));
#54405=CARTESIAN_POINT('Ctrl Pts',(-0.0782251060929565,0.0463398375912083,
-0.155589477191711));
#54406=CARTESIAN_POINT('Ctrl Pts',(-0.0813585786607769,-0.0405873064859364,
-0.150032710149149));
#54407=CARTESIAN_POINT('Ctrl Pts',(-0.0100267502373365,-0.0903659894557529,
-0.144475943106589));
#54408=CARTESIAN_POINT('Ctrl Pts',(0.0704822908518116,-0.0574351325482238,
-0.138919176064027));
#54409=CARTESIAN_POINT('Ctrl Pts',(0.0864808021551291,0.0280645438402883,
-0.133362409021466));
#54410=CARTESIAN_POINT('Ctrl Pts',(0.0233257803388205,0.0878775042030495,
-0.127805641978905));
#54411=CARTESIAN_POINT('Ctrl Pts',(-0.0611786960722008,0.0672585677921695,
-0.122248874936344));
#54412=CARTESIAN_POINT('Ctrl Pts',(-0.0896879702034033,-0.0149203120679575,
-0.116692107893783));
#54413=CARTESIAN_POINT('Ctrl Pts',(-0.0361082782663861,-0.0834430347416967,
-0.111135340851222));
#54414=CARTESIAN_POINT('Ctrl Pts',(0.0505203439252101,-0.0755926104834019,
-0.105578573808661));
#54415=CARTESIAN_POINT('Ctrl Pts',(0.0909090609484884,0.00144568087120341,
-0.1000218067661));
#54416=CARTESIAN_POINT('Ctrl Pts',(0.0480911874950899,0.0771607789491207,
-0.0944650397235385));
#54417=CARTESIAN_POINT('Ctrl Pts',(-0.0387432610833752,0.0822527097324212,
-0.0889082726809775));
#54418=CARTESIAN_POINT('Ctrl Pts',(-0.0901170244962536,0.0120609627886696,
-0.0833515056384163));
#54419=CARTESIAN_POINT('Ctrl Pts',(-0.0590091735361575,-0.069169851083726,
-0.0777947385958553));
#54420=CARTESIAN_POINT('Ctrl Pts',(0.0261082775077724,-0.087091385804074,
-0.0722379715532941));
#54421=CARTESIAN_POINT('Ctrl Pts',(0.0873293337077548,-0.025300517597168,
-0.0666812045107331));
#54422=CARTESIAN_POINT('Ctrl Pts',(0.068620590974884,0.0596471923669532,
-0.0611244374681719));
#54423=CARTESIAN_POINT('Ctrl Pts',(-0.0128954238312897,0.0900015126958784,
-0.055567670425611));
#54424=CARTESIAN_POINT('Ctrl Pts',(-0.0826072687683161,0.0379797595227237,
-0.0500109033830497));
#54425=CARTESIAN_POINT('Ctrl Pts',(-0.0767134573427241,-0.0488035925573516,
-0.0444541363404888));
#54426=CARTESIAN_POINT('Ctrl Pts',(-0.000601088932553975,-0.0909188044845557,
-0.0388973692979275));
#54427=CARTESIAN_POINT('Ctrl Pts',(0.076052321356028,-0.0498176186446183,
-0.0333406022553666));
#54428=CARTESIAN_POINT('Ctrl Pts',(0.0831143936316547,0.0368786114239041,
-0.0277838352128053));
#54429=CARTESIAN_POINT('Ctrl Pts',(0.0140713189020179,0.0898240214567205,
-0.0222270681702444));
#54430=CARTESIAN_POINT('Ctrl Pts',(-0.0677885288000042,0.0605498871972536,
-0.0166703011276831));
#54431=CARTESIAN_POINT('Ctrl Pts',(-0.0877227621557321,-0.0241321279134182,
-0.0111135340851222));
#54432=CARTESIAN_POINT('Ctrl Pts',(-0.0271300943677211,-0.0867515915827831,
-0.00555676704256098));
#54433=CARTESIAN_POINT('Ctrl Pts',(0.0294658500759831,-0.0755214844234609,
-0.00185225568085369));
#54434=CARTESIAN_POINT('Ctrl Pts',(0.0491442338326719,-0.0591802323922411,
0.));
#54435=CARTESIAN_POINT('Ctrl Pts',(-0.0701798155542591,-0.00332067636904823,
-0.568498003589195));
#54436=CARTESIAN_POINT('Ctrl Pts',(-0.0690756369919176,-0.0266565993052248,
-0.566645747908341));
#54437=CARTESIAN_POINT('Ctrl Pts',(-0.0417819951313892,-0.071736844313774,
-0.562941236546634));
#54438=CARTESIAN_POINT('Ctrl Pts',(0.037769664486587,-0.0740169623287969,
-0.557384469504073));
#54439=CARTESIAN_POINT('Ctrl Pts',(0.0825891842834973,-0.0084071600215922,
-0.551827702461512));
#54440=CARTESIAN_POINT('Ctrl Pts',(0.0518985613735119,0.0648242487603872,
-0.546270935418951));
#54441=CARTESIAN_POINT('Ctrl Pts',(-0.0263358835476263,0.0787620754562775,
-0.540714168376389));
#54442=CARTESIAN_POINT('Ctrl Pts',(-0.0804434647239304,0.0205909508341243,
-0.535157401333829));
#54443=CARTESIAN_POINT('Ctrl Pts',(-0.0609351020536189,-0.0564158842395974,
-0.529600634291267));
#54444=CARTESIAN_POINT('Ctrl Pts',(0.0143517189819161,-0.0817923957740036,
-0.524043867248707));
#54445=CARTESIAN_POINT('Ctrl Pts',(0.0764995244331497,-0.0323035885724571,
-0.518487100206145));
#54446=CARTESIAN_POINT('Ctrl Pts',(0.0686311175903372,0.0467502578079397,
-0.512930333163584));
#54447=CARTESIAN_POINT('Ctrl Pts',(-0.00205440178534356,0.0830156834418511,
-0.507373566121023));
#54448=CARTESIAN_POINT('Ctrl Pts',(-0.0708591021131913,0.0432986710962806,
-0.501816799078462));
#54449=CARTESIAN_POINT('Ctrl Pts',(-0.074808641219703,-0.0360482120029261,
-0.496260032035901));
#54450=CARTESIAN_POINT('Ctrl Pts',(-0.0102877256816388,-0.0824012648160085,
-0.49070326499334));
#54451=CARTESIAN_POINT('Ctrl Pts',(0.0636491956648538,-0.0533346105738538,
-0.485146497950778));
#54452=CARTESIAN_POINT('Ctrl Pts',(0.079329771278649,0.0245477329774338,
-0.479589730908218));
#54453=CARTESIAN_POINT('Ctrl Pts',(0.0224019386315129,0.0799622198593647,
-0.474032963865656));
#54454=CARTESIAN_POINT('Ctrl Pts',(-0.0550297706639658,0.0621894457294541,
-0.468476196823095));
#54455=CARTESIAN_POINT('Ctrl Pts',(-0.0820942284602035,-0.0125036368859546,
-0.462919429780535));
#54456=CARTESIAN_POINT('Ctrl Pts',(-0.0340200620447827,-0.0757524822944741,
-0.457362662737973));
#54457=CARTESIAN_POINT('Ctrl Pts',(0.0451917431893769,-0.0696671333103681,
-0.451805895695412));
#54458=CARTESIAN_POINT('Ctrl Pts',(0.0830407720544162,0.000182653050474542,
-0.446249128652851));
#54459=CARTESIAN_POINT('Ctrl Pts',(0.0448848334794573,0.0698652624083424,
-0.44069236161029));
#54460=CARTESIAN_POINT('Ctrl Pts',(-0.0343529759074532,0.0756020912738502,
-0.435135594567729));
#54461=CARTESIAN_POINT('Ctrl Pts',(-0.0821484380421907,0.012142376047441,
-0.429578827525167));
#54462=CARTESIAN_POINT('Ctrl Pts',(-0.0547556622234602,-0.0624309267915823,
-0.424022060482607));
#54463=CARTESIAN_POINT('Ctrl Pts',(0.0227534865001052,-0.0798628951185247,
-0.418465293440045));
#54464=CARTESIAN_POINT('Ctrl Pts',(0.0794369860064231,-0.0241985210353241,
-0.412908526397485));
#54465=CARTESIAN_POINT('Ctrl Pts',(0.0634139661397318,0.0536141032186852,
-0.407351759354923));
#54466=CARTESIAN_POINT('Ctrl Pts',(-0.0106501374650332,0.0823551925345891,
-0.401794992312362));
#54467=CARTESIAN_POINT('Ctrl Pts',(-0.0749664590282454,0.0357188071805889,
-0.396238225269801));
#54468=CARTESIAN_POINT('Ctrl Pts',(-0.0706680133513467,-0.0436100338742971,
-0.390681458227241));
#54469=CARTESIAN_POINT('Ctrl Pts',(-0.00168905121241881,-0.0830237934061215,
-0.385124691184679));
#54470=CARTESIAN_POINT('Ctrl Pts',(0.0688358537031139,-0.0464481260174393,
-0.379567924142118));
#54471=CARTESIAN_POINT('Ctrl Pts',(0.076357168202876,0.032640251677813,
-0.374011157099557));
#54472=CARTESIAN_POINT('Ctrl Pts',(0.0139908370653997,0.0818538920501867,
-0.368454390056996));
#54473=CARTESIAN_POINT('Ctrl Pts',(-0.0611809278776191,0.0561488844910692,
-0.362897623014435));
#54474=CARTESIAN_POINT('Ctrl Pts',(-0.0803554484503843,-0.0209476745700599,
-0.357340855971873));
#54475=CARTESIAN_POINT('Ctrl Pts',(-0.0259828058883404,-0.0788713950917863,
-0.351784088929313));
#54476=CARTESIAN_POINT('Ctrl Pts',(0.0521711943815237,-0.0646062662778276,
-0.346227321886752));
#54477=CARTESIAN_POINT('Ctrl Pts',(0.0825743150519032,0.00879122626628292,
-0.34067055484419));
#54478=CARTESIAN_POINT('Ctrl Pts',(0.0373994041514876,0.0741423477822878,
-0.33511378780163));
#54479=CARTESIAN_POINT('Ctrl Pts',(-0.0420061672868148,0.0716329887372305,
-0.329557020759068));
#54480=CARTESIAN_POINT('Ctrl Pts',(-0.0829646328014945,0.00355989742397316,
-0.324000253716507));
#54481=CARTESIAN_POINT('Ctrl Pts',(-0.0479878194926123,-0.0677714714751015,
-0.318443486673946));
#54482=CARTESIAN_POINT('Ctrl Pts',(0.0309109438118187,-0.0770734501512592,
-0.312886719631385));
#54483=CARTESIAN_POINT('Ctrl Pts',(0.081517758393159,-0.0158321897446498,
-0.307329952588824));
#54484=CARTESIAN_POINT('Ctrl Pts',(0.057513579064998,0.0598998446466287,
-0.301773185546262));
#54485=CARTESIAN_POINT('Ctrl Pts',(-0.0191312197050768,0.0808071754125344,
-0.296216418503702));
#54486=CARTESIAN_POINT('Ctrl Pts',(-0.0782657318206477,0.027753889603702,
-0.29065965146114));
#54487=CARTESIAN_POINT('Ctrl Pts',(-0.0657657417700864,-0.0507017788148143,
-0.28510288441858));
#54488=CARTESIAN_POINT('Ctrl Pts',(0.00692784848959868,-0.082751483858969,
-0.279546117376018));
#54489=CARTESIAN_POINT('Ctrl Pts',(0.0732805668748336,-0.0390609995271377,
-0.273989350333457));
#54490=CARTESIAN_POINT('Ctrl Pts',(0.0725615693964754,0.0403809585358808,
-0.268432583290896));
#54491=CARTESIAN_POINT('Ctrl Pts',(0.00542893495090355,0.0828633201775967,
-0.262875816248335));
#54492=CARTESIAN_POINT('Ctrl Pts',(-0.066672656450076,0.0495031316933198,
-0.257319049205774));
#54493=CARTESIAN_POINT('Ctrl Pts',(-0.0777505732262594,-0.029165930956239,
-0.251762282163213));
#54494=CARTESIAN_POINT('Ctrl Pts',(-0.0176654985292686,-0.08114020783353,
-0.246205515120651));
#54495=CARTESIAN_POINT('Ctrl Pts',(0.0585883279729262,-0.0588490525912939,
-0.240648748078091));
#54496=CARTESIAN_POINT('Ctrl Pts',(0.0812178464995143,0.017305044800213,
-0.235091981035529));
#54497=CARTESIAN_POINT('Ctrl Pts',(0.0295108723407657,0.0776203039110454,
-0.229535213992969));
#54498=CARTESIAN_POINT('Ctrl Pts',(-0.0492066030864478,0.0668918035206761,
-0.223978446950407));
#54499=CARTESIAN_POINT('Ctrl Pts',(-0.0828866089419013,-0.0050609508660535,
-0.218421679907846));
#54500=CARTESIAN_POINT('Ctrl Pts',(-0.0407027490968618,-0.0723815541523789,
-0.212864912865285));
#54501=CARTESIAN_POINT('Ctrl Pts',(0.0387352333446096,-0.0734532835433118,
-0.207308145822724));
#54502=CARTESIAN_POINT('Ctrl Pts',(0.0827199070086567,-0.00729521418719437,
-0.201751378780163));
#54503=CARTESIAN_POINT('Ctrl Pts',(0.0509932927315665,0.0655399669052933,
-0.196194611737602));
#54504=CARTESIAN_POINT('Ctrl Pts',(-0.0274060997034382,0.0783881934005274,
-0.190637844695041));
#54505=CARTESIAN_POINT('Ctrl Pts',(-0.0807214321943126,0.0194898319661148,
-0.18508107765248));
#54506=CARTESIAN_POINT('Ctrl Pts',(-0.0601546265529035,-0.0572470442016113,
-0.179524310609918));
#54507=CARTESIAN_POINT('Ctrl Pts',(0.0154700776838018,-0.0815872530607607,
-0.173967543567358));
#54508=CARTESIAN_POINT('Ctrl Pts',(0.0769354392874359,-0.0312528614255867,
-0.168410776524796));
#54509=CARTESIAN_POINT('Ctrl Pts',(0.0679838794080156,0.0476864268536628,
-0.162854009482235));
#54510=CARTESIAN_POINT('Ctrl Pts',(-0.0031914819124976,0.0829796216472279,
-0.157297242439674));
#54511=CARTESIAN_POINT('Ctrl Pts',(-0.0714457663817268,0.0423238187337744,
-0.151740475397113));
#54512=CARTESIAN_POINT('Ctrl Pts',(-0.0743076781160228,-0.0370698278607881,
-0.146183708354552));
#54513=CARTESIAN_POINT('Ctrl Pts',(-0.00915778694084917,-0.0825344661576702,
-0.140626941311991));
#54514=CARTESIAN_POINT('Ctrl Pts',(0.0643739783524676,-0.0524575455003868,
-0.13507017426943));
#54515=CARTESIAN_POINT('Ctrl Pts',(0.0789859866720714,0.0256323441791222,
-0.129513407226869));
#54516=CARTESIAN_POINT('Ctrl Pts',(0.0213042632473828,0.0802616442352845,
-0.123956640184308));
#54517=CARTESIAN_POINT('Ctrl Pts',(-0.0558766749631382,0.0614296376401015,
-0.118399873141747));
#54518=CARTESIAN_POINT('Ctrl Pts',(-0.0819152071048523,-0.0136272506819364,
-0.112843106099185));
#54519=CARTESIAN_POINT('Ctrl Pts',(-0.0329789723826125,-0.0762114858528055,
-0.107286339056624));
#54520=CARTESIAN_POINT('Ctrl Pts',(0.0461420235763678,-0.0690414146880683,
-0.101729572014063));
#54521=CARTESIAN_POINT('Ctrl Pts',(0.083030472630994,0.00132039166126336,
-0.096172804971502));
#54522=CARTESIAN_POINT('Ctrl Pts',(0.0439233887738163,0.0704736786177055,
-0.090616037928941));
#54523=CARTESIAN_POINT('Ctrl Pts',(-0.0353855957311171,0.0751243197653603,
-0.0850592708863799));
#54524=CARTESIAN_POINT('Ctrl Pts',(-0.0823070776219169,0.0110157054784169,
-0.0795025038438189));
#54525=CARTESIAN_POINT('Ctrl Pts',(-0.0538951730130365,-0.0631752805207342,
-0.0739457368012577));
#54526=CARTESIAN_POINT('Ctrl Pts',(0.0238456166902865,-0.0795436543943393,
-0.0683889697586967));
#54527=CARTESIAN_POINT('Ctrl Pts',(0.0797609806619091,-0.0231078608884972,
-0.0628322027161355));
#54528=CARTESIAN_POINT('Ctrl Pts',(0.0626736217646239,0.0544778982608371,
-0.0572754356735745));
#54529=CARTESIAN_POINT('Ctrl Pts',(-0.011777848371965,0.0822015765939713,
-0.0517186686310134));
#54530=CARTESIAN_POINT('Ctrl Pts',(-0.0754481511196702,0.0346882626515089,
-0.0461619015884522));
#54531=CARTESIAN_POINT('Ctrl Pts',(-0.07006512391469,-0.0445740536075221,
-0.0406051345458912));
#54532=CARTESIAN_POINT('Ctrl Pts',(-0.00054899586072548,-0.0830393717483792,
-0.0350483675033299));
#54533=CARTESIAN_POINT('Ctrl Pts',(0.0694612849477496,-0.0455001996308929,
-0.0294916004607691));
#54534=CARTESIAN_POINT('Ctrl Pts',(0.0759113262602619,0.0336825450021603,
-0.0239348334182077));
#54535=CARTESIAN_POINT('Ctrl Pts',(0.0128518350842712,0.0820394675443192,
-0.0183780663756468));
#54536=CARTESIAN_POINT('Ctrl Pts',(-0.0619136698421449,0.0553023614949671,
-0.0128212993330856));
#54537=CARTESIAN_POINT('Ctrl Pts',(-0.0801203128301351,-0.0220407291125593,
-0.00726453229052462));
#54538=CARTESIAN_POINT('Ctrl Pts',(-0.0247788783029195,-0.0792333082693582,
-0.00170776524796345));
#54539=CARTESIAN_POINT('Ctrl Pts',(0.0269122069104775,-0.068976452732553,
0.00199674611374385));
#54540=CARTESIAN_POINT('Ctrl Pts',(0.0448851733770188,-0.0540514071388779,
0.00384900179459754));
#54541=CARTESIAN_POINT('Ctrl Pts',(-0.0635205992758333,-0.00300558431647635,
-0.564649001794598));
#54542=CARTESIAN_POINT('Ctrl Pts',(-0.0625211939135715,-0.0241272102120953,
-0.562796746113744));
#54543=CARTESIAN_POINT('Ctrl Pts',(-0.0378173887851531,-0.0649298848248621,
-0.559092234752037));
#54544=CARTESIAN_POINT('Ctrl Pts',(0.0341857798241194,-0.0669936471985585,
-0.553535467709475));
#54545=CARTESIAN_POINT('Ctrl Pts',(0.0747524688966159,-0.00760942214740409,
-0.547978700666915));
#54546=CARTESIAN_POINT('Ctrl Pts',(0.0469740151632386,0.0586732110414563,
-0.542421933624353));
#54547=CARTESIAN_POINT('Ctrl Pts',(-0.0238369265036107,0.0712885064413299,
-0.536865166581792));
#54548=CARTESIAN_POINT('Ctrl Pts',(-0.0728103521893386,0.0186371184693627,
-0.531308399539231));
#54549=CARTESIAN_POINT('Ctrl Pts',(-0.0551530973515789,-0.0510626986872698,
-0.52575163249667));
#54550=CARTESIAN_POINT('Ctrl Pts',(0.012989914310403,-0.0740312859864097,
-0.520194865454109));
#54551=CARTESIAN_POINT('Ctrl Pts',(0.0692406441643183,-0.0292383684493435,
-0.514638098411548));
#54552=CARTESIAN_POINT('Ctrl Pts',(0.0621188540305847,0.0423142233818518,
-0.509081331368986));
#54553=CARTESIAN_POINT('Ctrl Pts',(-0.00185946388613005,0.0751384984396591,
-0.503524564326426));
#54554=CARTESIAN_POINT('Ctrl Pts',(-0.064135429750417,0.0391901505320498,
-0.497967797283864));
#54555=CARTESIAN_POINT('Ctrl Pts',(-0.0677102053312242,-0.0326276723750841,
-0.492411030241303));
#54556=CARTESIAN_POINT('Ctrl Pts',(-0.00931154485548331,-0.0745823807153317,
-0.486854263198743));
#54557=CARTESIAN_POINT('Ctrl Pts',(0.0576096562825884,-0.0482738006510584,
-0.481297496156181));
#54558=CARTESIAN_POINT('Ctrl Pts',(0.0718023347915276,0.0222184498103195,
-0.47574072911362));
#54559=CARTESIAN_POINT('Ctrl Pts',(0.0202762654130079,0.0723747716459273,
-0.470183962071059));
#54560=CARTESIAN_POINT('Ctrl Pts',(-0.0498081105369146,0.0562884189730116,
-0.464627195028498));
#54561=CARTESIAN_POINT('Ctrl Pts',(-0.0743044783987442,-0.0113171928687849,
-0.459070427985937));
#54562=CARTESIAN_POINT('Ctrl Pts',(-0.0307919693350411,-0.0685644872955918,
-0.453513660943375));
#54563=CARTESIAN_POINT('Ctrl Pts',(0.0409035929638406,-0.0630565643804312,
-0.447956893900815));
#54564=CARTESIAN_POINT('Ctrl Pts',(0.0751612064461215,0.000165321483593517,
-0.442400126858254));
#54565=CARTESIAN_POINT('Ctrl Pts',(0.0406258052759737,0.0632358934216658,
-0.436843359815692));
#54566=CARTESIAN_POINT('Ctrl Pts',(-0.0310932936958583,0.0684283665651463,
-0.431286592773132));
#54567=CARTESIAN_POINT('Ctrl Pts',(-0.0743535441465968,0.0109902113175206,
-0.42572982573057));
#54568=CARTESIAN_POINT('Ctrl Pts',(-0.049560011674442,-0.0565069864009689,
-0.42017305868801));
#54569=CARTESIAN_POINT('Ctrl Pts',(0.020594455637802,-0.0722848716225193,
-0.414616291645448));
#54570=CARTESIAN_POINT('Ctrl Pts',(0.0718993761374708,-0.0219023738608175,
-0.409059524602887));
#54571=CARTESIAN_POINT('Ctrl Pts',(0.0573967471963337,0.0485267728219418,
-0.403502757560326));
#54572=CARTESIAN_POINT('Ctrl Pts',(-0.00963956814086993,0.0745406801365732,
-0.397945990517764));
#54573=CARTESIAN_POINT('Ctrl Pts',(-0.0678530481371775,0.0323295240890841,
-0.392389223475204));
#54574=CARTESIAN_POINT('Ctrl Pts',(-0.0639624730025055,-0.0394719687456726,
-0.386832456432642));
#54575=CARTESIAN_POINT('Ctrl Pts',(-0.00152878066682028,-0.0751458388663401,
-0.381275689390082));
#54576=CARTESIAN_POINT('Ctrl Pts',(0.0623041631607716,-0.0420407602465988,
-0.375718922347521));
#54577=CARTESIAN_POINT('Ctrl Pts',(0.0691117958197301,0.0295430862950298,
-0.370162155304959));
#54578=CARTESIAN_POINT('Ctrl Pts',(0.0126632757260182,0.0740869470092486,
-0.364605388262398));
#54579=CARTESIAN_POINT('Ctrl Pts',(-0.0553755972760191,0.0508210339878241,
-0.359048621219837));
#54580=CARTESIAN_POINT('Ctrl Pts',(-0.0727306875963563,-0.0189599934342466,
-0.353491854177276));
#54581=CARTESIAN_POINT('Ctrl Pts',(-0.0235173516467703,-0.0713874529647044,
-0.347935087134715));
#54582=CARTESIAN_POINT('Ctrl Pts',(0.0472207785939286,-0.0584759124618787,
-0.342378320092153));
#54583=CARTESIAN_POINT('Ctrl Pts',(0.0747390105753852,0.00795704514743341,
-0.336821553049593));
#54584=CARTESIAN_POINT('Ctrl Pts',(0.0338506527197245,0.0671071350879659,
-0.331264786007032));
#54585=CARTESIAN_POINT('Ctrl Pts',(-0.0380202897124528,0.0648358838872972,
-0.325708018964471));
#54586=CARTESIAN_POINT('Ctrl Pts',(-0.0750922918880565,0.00322210618459649,
-0.320151251921909));
#54587=CARTESIAN_POINT('Ctrl Pts',(-0.043434355420249,-0.0613407779417036,
-0.314594484879349));
#54588=CARTESIAN_POINT('Ctrl Pts',(0.0279778688445018,-0.0697601112684447,
-0.309037717836787));
#54589=CARTESIAN_POINT('Ctrl Pts',(0.0737827083736445,-0.0143299062912367,
-0.303480950794226));
#54590=CARTESIAN_POINT('Ctrl Pts',(0.0520562355408607,0.0542160733600317,
-0.297924183751665));
#54591=CARTESIAN_POINT('Ctrl Pts',(-0.0173158981816449,0.0731395511295278,
-0.292367416709104));
#54592=CARTESIAN_POINT('Ctrl Pts',(-0.0708392598177398,0.0251203809234781,
-0.286810649666543));
#54593=CARTESIAN_POINT('Ctrl Pts',(-0.0595253677437465,-0.045890792804632,
-0.281253882623981));
#54594=CARTESIAN_POINT('Ctrl Pts',(0.00627047940032424,-0.0748993682039843,
-0.275697115581421));
#54595=CARTESIAN_POINT('Ctrl Pts',(0.0663271267728453,-0.0353545827768454,
-0.27014034853886));
#54596=CARTESIAN_POINT('Ctrl Pts',(0.0656763534651288,0.0365492936291439,
-0.264583581496299));
#54597=CARTESIAN_POINT('Ctrl Pts',(0.00491379464005916,0.075000592607667,
-0.259026814453737));
#54598=CARTESIAN_POINT('Ctrl Pts',(-0.0603462271818922,0.0448058828077,
-0.253470047411177));
#54599=CARTESIAN_POINT('Ctrl Pts',(-0.0703729835475725,-0.0263984366180838,
-0.247913280368615));
#54600=CARTESIAN_POINT('Ctrl Pts',(-0.0159892562302031,-0.073440982798917,
-0.242356513326054));
#54601=CARTESIAN_POINT('Ctrl Pts',(0.0530290037672167,-0.0532649887705087,
-0.236799746283493));
#54602=CARTESIAN_POINT('Ctrl Pts',(0.073511254493867,0.0156630052034671,
-0.231242979240932));
#54603=CARTESIAN_POINT('Ctrl Pts',(0.0267106472342993,0.0702550752158925,
-0.225686212198371));
#54604=CARTESIAN_POINT('Ctrl Pts',(-0.0445374911816733,0.0605445798441793,
-0.22012944515581));
#54605=CARTESIAN_POINT('Ctrl Pts',(-0.0750216715497152,-0.00458072779727913,
-0.214572678113249));
#54606=CARTESIAN_POINT('Ctrl Pts',(-0.0368405501551592,-0.0655134194919708,
-0.209015911070687));
#54607=CARTESIAN_POINT('Ctrl Pts',(0.0350597278677169,-0.066483454716998,
-0.203459144028127));
#54608=CARTESIAN_POINT('Ctrl Pts',(0.074870787615118,-0.00660298653332633,
-0.197902376985565));
#54609=CARTESIAN_POINT('Ctrl Pts',(0.0461546455740219,0.0593210161848294,
-0.192345609943004));
#54610=CARTESIAN_POINT('Ctrl Pts',(-0.0248055920812409,0.0709501012738018,
-0.186788842900443));
#54611=CARTESIAN_POINT('Ctrl Pts',(-0.0730619439063931,0.0176404824734215,
-0.181232075857882));
#54612=CARTESIAN_POINT('Ctrl Pts',(-0.0544466795427829,-0.0518149916145772,
-0.175675308815321));
#54613=CARTESIAN_POINT('Ctrl Pts',(0.0140021542883522,-0.0738456088372273,
-0.17011854177276));
#54614=CARTESIAN_POINT('Ctrl Pts',(0.0696351959675514,-0.0282873426092572,
-0.164561774730199));
#54615=CARTESIAN_POINT('Ctrl Pts',(0.0615330309290195,0.0431615613000007,
-0.159005007687638));
#54616=CARTESIAN_POINT('Ctrl Pts',(-0.00288864885236336,0.0751058584734902,
-0.153448240645077));
#54617=CARTESIAN_POINT('Ctrl Pts',(-0.0646664266704969,0.0383077998763405,
-0.147891473602516));
#54618=CARTESIAN_POINT('Ctrl Pts',(-0.0672567775712689,-0.0335523492356398,
-0.142334706559954));
#54619=CARTESIAN_POINT('Ctrl Pts',(-0.00828882364436172,-0.0747029428595875,
-0.136777939517393));
#54620=CARTESIAN_POINT('Ctrl Pts',(0.0582656658531234,-0.0474799584525497,
-0.131221172474832));
#54621=CARTESIAN_POINT('Ctrl Pts',(0.0714911711890138,0.023200144517956,
-0.125664405432271));
#54622=CARTESIAN_POINT('Ctrl Pts',(0.019282746155945,0.0726457842675196,
-0.12010763838971));
#54623=CARTESIAN_POINT('Ctrl Pts',(-0.0505746538540758,0.0556007074880334,
-0.114550871347149));
#54624=CARTESIAN_POINT('Ctrl Pts',(-0.0741424440063013,-0.0123341892959154,
-0.108994104304588));
#54625=CARTESIAN_POINT('Ctrl Pts',(-0.0298496664988389,-0.0689799369639143,
-0.103437337262027));
#54626=CARTESIAN_POINT('Ctrl Pts',(0.0417637032275256,-0.0624902188927347,
-0.0978805702194657));
#54627=CARTESIAN_POINT('Ctrl Pts',(0.0751518843134995,0.00119510245132327,
-0.0923238031769045));
#54628=CARTESIAN_POINT('Ctrl Pts',(0.0397555900525427,0.0637865782862904,
-0.0867670361343434));
#54629=CARTESIAN_POINT('Ctrl Pts',(-0.032027930378859,0.0679959297982993,
-0.0812102690917824));
#54630=CARTESIAN_POINT('Ctrl Pts',(-0.0744971307475801,0.00997044816816438,
-0.0756535020492212));
#54631=CARTESIAN_POINT('Ctrl Pts',(-0.0487811724899154,-0.0571807099577425,
-0.0700967350066602));
#54632=CARTESIAN_POINT('Ctrl Pts',(0.0215829558728007,-0.0719959229846046,
-0.064539967964099));
#54633=CARTESIAN_POINT('Ctrl Pts',(0.0721926276160632,-0.0209152041798264,
-0.058983200921538));
#54634=CARTESIAN_POINT('Ctrl Pts',(0.0567266525543639,0.0493086041547209,
-0.0534264338789769));
#54635=CARTESIAN_POINT('Ctrl Pts',(-0.0106602729126405,0.0744016404920643,
-0.0478696668364159));
#54636=CARTESIAN_POINT('Ctrl Pts',(-0.0682890334710242,0.031396765780294,
-0.0423128997938546));
#54637=CARTESIAN_POINT('Ctrl Pts',(-0.063416790486656,-0.0403445146576926,
-0.0367561327512936));
#54638=CARTESIAN_POINT('Ctrl Pts',(-0.000496902788896909,-0.0751599390122028,
-0.0311993657087325));
#54639=CARTESIAN_POINT('Ctrl Pts',(0.062870248539471,-0.0411827806171674,
-0.0256425986661715));
#54640=CARTESIAN_POINT('Ctrl Pts',(0.0687082588888692,0.0304864785804164,
-0.0200858316236103));
#54641=CARTESIAN_POINT('Ctrl Pts',(0.0116323512665244,0.074254913631918,
-0.0145290645810492));
#54642=CARTESIAN_POINT('Ctrl Pts',(-0.0560388108842856,0.0500548357926805,
-0.0089722975384881));
#54643=CARTESIAN_POINT('Ctrl Pts',(-0.0725178635045378,-0.0199493303117004,
-0.00341553049592708));
#54644=CARTESIAN_POINT('Ctrl Pts',(-0.0224276622381181,-0.0717150249559334,
0.00214123654663408));
#54645=CARTESIAN_POINT('Ctrl Pts',(0.0243585637449721,-0.0624314210416452,
0.00584574790834138));
#54646=CARTESIAN_POINT('Ctrl Pts',(0.0406261129213658,-0.0489225818855146,
0.00769800358919507));
#54647=CARTESIAN_POINT('Ctrl Pts',(-0.0568613829974076,-0.00269049226390446,
-0.5608));
#54648=CARTESIAN_POINT('Ctrl Pts',(-0.0559667508352254,-0.0215978211189658,
-0.558947744319147));
#54649=CARTESIAN_POINT('Ctrl Pts',(-0.033852782438917,-0.0581229253359501,
-0.555243232957439));
#54650=CARTESIAN_POINT('Ctrl Pts',(0.0306018951616518,-0.0599703320683201,
-0.549686465914878));
#54651=CARTESIAN_POINT('Ctrl Pts',(0.0669157535097345,-0.00681168427321597,
-0.544129698872316));
#54652=CARTESIAN_POINT('Ctrl Pts',(0.0420494689529653,0.0525221733225254,
-0.538572931829757));
#54653=CARTESIAN_POINT('Ctrl Pts',(-0.0213379694595951,0.0638149374263822,
-0.533016164787193));
#54654=CARTESIAN_POINT('Ctrl Pts',(-0.0651772396547469,0.0166832861046011,
-0.527459397744635));
#54655=CARTESIAN_POINT('Ctrl Pts',(-0.0493710926495389,-0.0457095131349423,
-0.521902630702072));
#54656=CARTESIAN_POINT('Ctrl Pts',(0.0116281096388898,-0.0662701761988158,
-0.516345863659512));
#54657=CARTESIAN_POINT('Ctrl Pts',(0.061981763895487,-0.0261731483262298,
-0.51078909661695));
#54658=CARTESIAN_POINT('Ctrl Pts',(0.0556065904708322,0.0378781889557639,
-0.505232329574389));
#54659=CARTESIAN_POINT('Ctrl Pts',(-0.00166452598691655,0.0672613134374671,
-0.499675562531828));
#54660=CARTESIAN_POINT('Ctrl Pts',(-0.0574117573876428,0.035081629967819,
-0.494118795489267));
#54661=CARTESIAN_POINT('Ctrl Pts',(-0.0606117694427453,-0.0292071327472421,
-0.488562028446706));
#54662=CARTESIAN_POINT('Ctrl Pts',(-0.00833536402932787,-0.066763496614655,
-0.483005261404145));
#54663=CARTESIAN_POINT('Ctrl Pts',(0.0515701169003231,-0.0432129907282631,
-0.477448494361583));
#54664=CARTESIAN_POINT('Ctrl Pts',(0.064274898304406,0.019889166643205,
-0.471891727319023));
#54665=CARTESIAN_POINT('Ctrl Pts',(0.0181505921945029,0.06478732343249,
-0.466334960276461));
#54666=CARTESIAN_POINT('Ctrl Pts',(-0.0445864504098636,0.050387392216569,
-0.4607781932339));
#54667=CARTESIAN_POINT('Ctrl Pts',(-0.0665147283372848,-0.0101307488516152,
-0.45522142619134));
#54668=CARTESIAN_POINT('Ctrl Pts',(-0.0275638766252995,-0.0613764922967096,
-0.449664659148778));
#54669=CARTESIAN_POINT('Ctrl Pts',(0.0366154427383043,-0.0564459954504943,
-0.444107892106218));
#54670=CARTESIAN_POINT('Ctrl Pts',(0.0672816408378267,0.000147989916712509,
-0.438551125063656));
#54671=CARTESIAN_POINT('Ctrl Pts',(0.03636677707249,0.0566065244349891,
-0.432994358021095));
#54672=CARTESIAN_POINT('Ctrl Pts',(-0.0278336114842633,0.0612546418564424,
-0.427437590978534));
#54673=CARTESIAN_POINT('Ctrl Pts',(-0.0665586502510029,0.00983804658760028,
-0.421880823935972));
#54674=CARTESIAN_POINT('Ctrl Pts',(-0.0443643611254238,-0.0505830460103554,
-0.416324056893412));
#54675=CARTESIAN_POINT('Ctrl Pts',(0.0184354247754988,-0.0647068481265139,
-0.41076728985085));
#54676=CARTESIAN_POINT('Ctrl Pts',(0.0643617662685185,-0.0196062266863109,
-0.40521052280829));
#54677=CARTESIAN_POINT('Ctrl Pts',(0.0513795282529356,0.0434394424251984,
-0.399653755765729));
#54678=CARTESIAN_POINT('Ctrl Pts',(-0.00862899881670666,0.0667261677385573,
-0.394096988723167));
#54679=CARTESIAN_POINT('Ctrl Pts',(-0.0607396372461095,0.0289402409975793,
-0.388540221680607));
#54680=CARTESIAN_POINT('Ctrl Pts',(-0.0572569326536643,-0.0353339036170481,
-0.382983454638045));
#54681=CARTESIAN_POINT('Ctrl Pts',(-0.00136851012122178,-0.0672678843265587,
-0.377426687595484));
#54682=CARTESIAN_POINT('Ctrl Pts',(0.0557724726184293,-0.0376333944757582,
-0.371869920552923));
#54683=CARTESIAN_POINT('Ctrl Pts',(0.0618664234365842,0.0264459209122466,
-0.366313153510362));
#54684=CARTESIAN_POINT('Ctrl Pts',(0.0113357143866367,0.0663200019683107,
-0.360756386467801));
#54685=CARTESIAN_POINT('Ctrl Pts',(-0.0495702666744188,0.0454931834845789,
-0.35519961942524));
#54686=CARTESIAN_POINT('Ctrl Pts',(-0.0651059267423285,-0.0169723122984332,
-0.349642852382678));
#54687=CARTESIAN_POINT('Ctrl Pts',(-0.0210518974052001,-0.0639035108376226,
-0.344086085340117));
#54688=CARTESIAN_POINT('Ctrl Pts',(0.0422703628063335,-0.0523455586459296,
-0.338529318297556));
#54689=CARTESIAN_POINT('Ctrl Pts',(0.0669037060988672,0.00712286402858384,
-0.332972551254995));
#54690=CARTESIAN_POINT('Ctrl Pts',(0.0303019012879613,0.0600719223936441,
-0.327415784212435));
#54691=CARTESIAN_POINT('Ctrl Pts',(-0.0340344121380907,0.0580387790373639,
-0.321859017169872));
#54692=CARTESIAN_POINT('Ctrl Pts',(-0.0672199509746185,0.00288431494521986,
-0.316302250127312));
#54693=CARTESIAN_POINT('Ctrl Pts',(-0.0388808913478858,-0.0549100844083057,
-0.310745483084751));
#54694=CARTESIAN_POINT('Ctrl Pts',(0.0250447938771848,-0.0624467723856301,
-0.30518871604219));
#54695=CARTESIAN_POINT('Ctrl Pts',(0.0660476583541301,-0.0128276228378236,
-0.299631948999629));
#54696=CARTESIAN_POINT('Ctrl Pts',(0.0465988920167232,0.0485323020734347,
-0.294075181957067));
#54697=CARTESIAN_POINT('Ctrl Pts',(-0.0155005766582128,0.0654719268465212,
-0.288518414914507));
#54698=CARTESIAN_POINT('Ctrl Pts',(-0.0634127878148319,0.0224868722432543,
-0.282961647871945));
#54699=CARTESIAN_POINT('Ctrl Pts',(-0.0532849937174065,-0.0410798067944498,
-0.277404880829384));
#54700=CARTESIAN_POINT('Ctrl Pts',(0.0056131103110498,-0.0670472525489997,
-0.271848113786823));
#54701=CARTESIAN_POINT('Ctrl Pts',(0.0593736866708568,-0.0316481660265529,
-0.266291346744262));
#54702=CARTESIAN_POINT('Ctrl Pts',(0.0587911375337822,0.0327176287224069,
-0.2607345797017));
#54703=CARTESIAN_POINT('Ctrl Pts',(0.00439865432921479,0.0671378650377374,
-0.25517781265914));
#54704=CARTESIAN_POINT('Ctrl Pts',(-0.0540197979137084,0.0401086339220801,
-0.249621045616579));
#54705=CARTESIAN_POINT('Ctrl Pts',(-0.0629953938688856,-0.0236309422799287,
-0.244064278574018));
#54706=CARTESIAN_POINT('Ctrl Pts',(-0.0143130139311376,-0.0657417577643039,
-0.238507511531456));
#54707=CARTESIAN_POINT('Ctrl Pts',(0.0474696795615072,-0.0476809249497236,
-0.232950744488896));
#54708=CARTESIAN_POINT('Ctrl Pts',(0.0658046624882197,0.0140209656067212,
-0.227393977446334));
#54709=CARTESIAN_POINT('Ctrl Pts',(0.0239104221278329,0.0628898465207396,
-0.221837210403774));
#54710=CARTESIAN_POINT('Ctrl Pts',(-0.0398683792768989,0.0541973561676825,
-0.216280443361212));
#54711=CARTESIAN_POINT('Ctrl Pts',(-0.0671567341575291,-0.00410050472850469,
-0.210723676318652));
#54712=CARTESIAN_POINT('Ctrl Pts',(-0.0329783512134566,-0.0586452848315629,
-0.20516690927609));
#54713=CARTESIAN_POINT('Ctrl Pts',(0.0313842223908242,-0.059513625890684,
-0.199610142233529));
#54714=CARTESIAN_POINT('Ctrl Pts',(0.0670216682215793,-0.00591075887945832,
-0.194053375190967));
#54715=CARTESIAN_POINT('Ctrl Pts',(0.0413159984164774,0.0531020654643655,
-0.188496608148407));
#54716=CARTESIAN_POINT('Ctrl Pts',(-0.0222050844590437,0.0635120091470762,
-0.182939841105846));
#54717=CARTESIAN_POINT('Ctrl Pts',(-0.0654024556184737,0.0157911329807281,
-0.177383074063285));
#54718=CARTESIAN_POINT('Ctrl Pts',(-0.0487387325326623,-0.046382939027543,
-0.171826307020724));
#54719=CARTESIAN_POINT('Ctrl Pts',(0.0125342308929026,-0.066103964613694,
-0.166269539978162));
#54720=CARTESIAN_POINT('Ctrl Pts',(0.0623349526476669,-0.0253218237929275,
-0.160712772935602));
#54721=CARTESIAN_POINT('Ctrl Pts',(0.0550821824500234,0.0386366957463386,
-0.15515600589304));
#54722=CARTESIAN_POINT('Ctrl Pts',(-0.00258581579222903,0.0672320952997525,
-0.149599238850479));
#54723=CARTESIAN_POINT('Ctrl Pts',(-0.0578870869592672,0.0342917810189067,
-0.144042471807918));
#54724=CARTESIAN_POINT('Ctrl Pts',(-0.0602058770265148,-0.0300348706104915,
-0.138485704765357));
#54725=CARTESIAN_POINT('Ctrl Pts',(-0.00741986034787437,-0.0668714195615047,
-0.132928937722796));
#54726=CARTESIAN_POINT('Ctrl Pts',(0.0521573533537793,-0.0425023714047127,
-0.127372170680235));
#54727=CARTESIAN_POINT('Ctrl Pts',(0.0639963557059561,0.0207679448567898,
-0.121815403637674));
#54728=CARTESIAN_POINT('Ctrl Pts',(0.0172612290645072,0.0650299242997547,
-0.116258636595113));
#54729=CARTESIAN_POINT('Ctrl Pts',(-0.0452726327450133,0.0497717773359655,
-0.110701869552551));
#54730=CARTESIAN_POINT('Ctrl Pts',(-0.0663696809077504,-0.0110411279098944,
-0.10514510250999));
#54731=CARTESIAN_POINT('Ctrl Pts',(-0.0267203606150653,-0.061748388075023,
-0.0995883354674292));
#54732=CARTESIAN_POINT('Ctrl Pts',(0.0373853828786833,-0.055939023097401,
-0.0940315684248681));
#54733=CARTESIAN_POINT('Ctrl Pts',(0.0672732959960052,0.00106981324138322,
-0.088474801382307));
#54734=CARTESIAN_POINT('Ctrl Pts',(0.035587791331269,0.0570994779548752,
-0.0829180343397459));
#54735=CARTESIAN_POINT('Ctrl Pts',(-0.0286702650266008,0.0608675398312384,
-0.0773612672971849));
#54736=CARTESIAN_POINT('Ctrl Pts',(-0.0666871838732434,0.00892519085791185,
-0.0718045002546237));
#54737=CARTESIAN_POINT('Ctrl Pts',(-0.0436671719667944,-0.0511861393947508,
-0.0662477332120627));
#54738=CARTESIAN_POINT('Ctrl Pts',(0.0193202950553148,-0.0644481915748698,
-0.0606909661695014));
#54739=CARTESIAN_POINT('Ctrl Pts',(0.0646242745702175,-0.0187225474711557,
-0.0551341991269405));
#54740=CARTESIAN_POINT('Ctrl Pts',(0.0507796833441037,0.0441393100486048,
-0.0495774320843793));
#54741=CARTESIAN_POINT('Ctrl Pts',(-0.00954269745331579,0.0666017043901573,
-0.0440206650418183));
#54742=CARTESIAN_POINT('Ctrl Pts',(-0.0611299158223783,0.0281052689090792,
-0.0384638979992571));
#54743=CARTESIAN_POINT('Ctrl Pts',(-0.0567684570586219,-0.036114975707863,
-0.0329071309566961));
#54744=CARTESIAN_POINT('Ctrl Pts',(-0.000444809717068389,-0.0672805062760264,
-0.0273503639141349));
#54745=CARTESIAN_POINT('Ctrl Pts',(0.0562792121311924,-0.036865361603442,
-0.021793596871574));
#54746=CARTESIAN_POINT('Ctrl Pts',(0.0615051915174765,0.0272904121586725,
-0.0162368298290127));
#54747=CARTESIAN_POINT('Ctrl Pts',(0.0104128674487777,0.0664703597195168,
-0.0106800627864517));
#54748=CARTESIAN_POINT('Ctrl Pts',(-0.0501639519264263,0.044807310090394,
-0.00512329574389055));
#54749=CARTESIAN_POINT('Ctrl Pts',(-0.0649154141789406,-0.0178579315108415,
0.00043347129867045));
#54750=CARTESIAN_POINT('Ctrl Pts',(-0.0200764461733167,-0.0641967416425085,
0.00599023834123162));
#54751=CARTESIAN_POINT('Ctrl Pts',(0.0218049205794665,-0.0558863893507373,
0.00969474970293892));
#54752=CARTESIAN_POINT('Ctrl Pts',(0.0363670524657127,-0.0437937566321514,
0.0115470053837926));
#54753=CARTESIAN_POINT('',(0.0491442338326711,-0.0591802323922418,0.));
#54754=CARTESIAN_POINT('Ctrl Pts',(-0.05597698479429,-0.0108401358572846,
1.04083408558608E-17));
#54755=CARTESIAN_POINT('Ctrl Pts',(-0.0559515023807956,-0.0123446174890954,
1.17559405793022E-17));
#54756=CARTESIAN_POINT('Ctrl Pts',(-0.0558623774955055,-0.0138447025863335,
3.0034649799714E-17));
#54757=CARTESIAN_POINT('Ctrl Pts',(-0.055708865632993,-0.0153365024293318,
4.68375338513738E-17));
#54758=CARTESIAN_POINT('Ctrl Pts',(-0.0553750133694311,-0.0185808168830483,
8.34714469153916E-17));
#54759=CARTESIAN_POINT('Ctrl Pts',(-0.0547373288205537,-0.0217858319569694,
3.70891418926431E-17));
#54760=CARTESIAN_POINT('Ctrl Pts',(-0.0538263802290202,-0.0249261037145957,
4.5102810375397E-17));
#54761=CARTESIAN_POINT('Ctrl Pts',(-0.0532138536290939,-0.0270376388774144,
5.04912429985968E-17));
#54762=CARTESIAN_POINT('Ctrl Pts',(-0.0524775926510349,-0.0291185320549929,
-1.9163422263778E-17));
#54763=CARTESIAN_POINT('Ctrl Pts',(-0.0516300698525238,-0.0311521551872357,
-1.21430643318376E-17));
#54764=CARTESIAN_POINT('Ctrl Pts',(-0.0501225335147105,-0.0347694747149932,
3.44440081553474E-19));
#54765=CARTESIAN_POINT('Ctrl Pts',(-0.0482617497084152,-0.0382452636414351,
1.86132677700906E-16));
#54766=CARTESIAN_POINT('Ctrl Pts',(-0.0460910809893396,-0.0415384799097066,
1.2490009027033E-16));
#54767=CARTESIAN_POINT('Ctrl Pts',(-0.0448562377753026,-0.0434119144534002,
9.00662879484486E-17));
#54768=CARTESIAN_POINT('Ctrl Pts',(-0.0435260602506697,-0.0452182508027399,
8.80667632144303E-17));
#54769=CARTESIAN_POINT('Ctrl Pts',(-0.0421096187004071,-0.046950364248589,
9.36750677027476E-17));
#54770=CARTESIAN_POINT('Ctrl Pts',(-0.0397651997051909,-0.0498172666375831,
1.02957636101656E-16));
#54771=CARTESIAN_POINT('Ctrl Pts',(-0.0371848385423227,-0.0524812110416646,
9.99035557290718E-17));
#54772=CARTESIAN_POINT('Ctrl Pts',(-0.0344006017048867,-0.0549099186113641,
1.37910516340156E-16));
#54773=CARTESIAN_POINT('Ctrl Pts',(-0.0327159861626315,-0.0563794195045698,
1.60906805915247E-16));
#54774=CARTESIAN_POINT('Ctrl Pts',(-0.030956531645651,-0.0577627741542382,
6.77527425510591E-17));
#54775=CARTESIAN_POINT('Ctrl Pts',(-0.0291277574335744,-0.0590520230017192,
8.41340885848751E-17));
#54776=CARTESIAN_POINT('Ctrl Pts',(-0.0273557380977418,-0.0603012608088524,
1.00007049679358E-16));
#54777=CARTESIAN_POINT('Ctrl Pts',(-0.0255258512225868,-0.0614569060963195,
-2.78362784928054E-17));
#54778=CARTESIAN_POINT('Ctrl Pts',(-0.0236467459224507,-0.0625118270565618,
-8.67361737988404E-19));
#54779=CARTESIAN_POINT('Ctrl Pts',(-0.0225129729697565,-0.063148321909653,
1.54045461629985E-17));
#54780=CARTESIAN_POINT('Ctrl Pts',(-0.0213610269805812,-0.0637483119177658,
2.74020614788251E-17));
#54781=CARTESIAN_POINT('Ctrl Pts',(-0.0201922068122268,-0.0643104725864732,
2.08166817117217E-17));
#54782=CARTESIAN_POINT('Ctrl Pts',(-0.0159953557649841,-0.06632900773419,
-2.89476499819983E-18));
#54783=CARTESIAN_POINT('Ctrl Pts',(-0.0115821440144441,-0.0678613924765087,
8.36577011636678E-17));
#54784=CARTESIAN_POINT('Ctrl Pts',(-0.00702730608058084,-0.0689290076177083,
3.29597460435593E-17));
#54785=CARTESIAN_POINT('Ctrl Pts',(-0.00486576782889167,-0.0694356537375689,
8.90058721821139E-18));
#54786=CARTESIAN_POINT('Ctrl Pts',(-0.00267298950544152,-0.0698366915944207,
1.55243141773906E-16));
#54787=CARTESIAN_POINT('Ctrl Pts',(-0.000469913444744201,-0.0701325044915826,
1.50487261540988E-16));
#54788=CARTESIAN_POINT('Ctrl Pts',(0.00411297771785086,-0.0707478615082424,
1.40593966489296E-16));
#54789=CARTESIAN_POINT('Ctrl Pts',(0.00875406260761827,-0.0709126569904891,
-5.24987388074468E-17));
#54790=CARTESIAN_POINT('Ctrl Pts',(0.0133848262570198,-0.0706465207975322,
-8.15320033709099E-17));
#54791=CARTESIAN_POINT('Ctrl Pts',(0.01601004384827,-0.0704956460243166,
-9.79911972823228E-17));
#54792=CARTESIAN_POINT('Ctrl Pts',(0.0186321482126508,-0.0702059750708208,
-2.51203942901452E-17));
#54793=CARTESIAN_POINT('Ctrl Pts',(0.021239506109343,-0.0697786235236676,
-9.54097911787244E-18));
#54794=CARTESIAN_POINT('Ctrl Pts',(0.0234844735095893,-0.0694106685555288,
3.87309005192856E-18));
#54795=CARTESIAN_POINT('Ctrl Pts',(0.0257136024412654,-0.0689411634638083,
9.07880977736139E-19));
#54796=CARTESIAN_POINT('Ctrl Pts',(0.0279116068143838,-0.0683739194742597,
-6.28837260041593E-18));
#54797=CARTESIAN_POINT('Ctrl Pts',(0.0340160087394049,-0.0667985425805166,
-2.62741491223654E-17));
#54798=CARTESIAN_POINT('Ctrl Pts',(0.0398983402063176,-0.0644702353768579,
1.18194476211714E-16));
#54799=CARTESIAN_POINT('Ctrl Pts',(0.0454040549742523,-0.061410347827305,
1.31080042653497E-16));
#54800=CARTESIAN_POINT('Ctrl Pts',(0.0466714005203764,-0.0607060006133608,
1.34046136235822E-16));
#54801=CARTESIAN_POINT('Ctrl Pts',(0.0479187804398171,-0.0599626729111359,
-2.46165589825557E-18));
#54802=CARTESIAN_POINT('Ctrl Pts',(0.0491442338326719,-0.0591802323922411,
0.));
#54803=CARTESIAN_POINT('Ctrl Pts',(0.0491442338326711,-0.0591802323922418,
-7.97972798949331E-17));
#54804=CARTESIAN_POINT('Ctrl Pts',(0.0294658500759823,-0.0755214844234611,
-0.00185225568085374));
#54805=CARTESIAN_POINT('Ctrl Pts',(0.00116787785413063,-0.0811365380031219,
-0.00370451136170736));
#54806=CARTESIAN_POINT('Ctrl Pts',(-0.0230798862214635,-0.0735074875147251,
-0.00555676704256102));
#54807=CARTESIAN_POINT('Ctrl Pts',(-0.047327650297058,-0.0658784370263282,
-0.00740902272341471));
#54808=CARTESIAN_POINT('Ctrl Pts',(-0.0675252062263949,-0.0450052824698734,
-0.00926127840426843));
#54809=CARTESIAN_POINT('Ctrl Pts',(-0.0743016119651088,-0.0204550360065341,
-0.0111135340851221));
#54810=CARTESIAN_POINT('Ctrl Pts',(-0.0761269997977368,-0.0138418367811431,
-0.0116124836924973));
#54811=CARTESIAN_POINT('Ctrl Pts',(-0.0769785170734933,-0.00696181902737242,
-0.0121114332998725));
#54812=CARTESIAN_POINT('Ctrl Pts',(-0.0769167618896329,-6.73610264414135E-5,
-0.0126103829072477));
#54813=CARTESIAN_POINT('Origin',(0.,0.,-0.2904));
#54814=CARTESIAN_POINT('Origin',(0.,0.,0.));
#54815=CARTESIAN_POINT('Origin',(-0.0288,-0.1152,0.0585));
#54816=CARTESIAN_POINT('',(0.0288,-0.1152,0.13));
#54817=CARTESIAN_POINT('',(-0.0288,-0.1152,0.13));
#54818=CARTESIAN_POINT('',(-0.0144,-0.1152,0.13));
#54819=CARTESIAN_POINT('',(0.0288,-0.1152,0.0585));
#54820=CARTESIAN_POINT('',(0.0288,-0.1152,0.0585));
#54821=CARTESIAN_POINT('',(-0.0288,-0.1152,0.0585));
#54822=CARTESIAN_POINT('',(-0.0288,-0.1152,0.0585));
#54823=CARTESIAN_POINT('',(-0.0288,-0.1152,0.0585));
#54824=CARTESIAN_POINT('Origin',(0.0288,-0.1152,0.0585));
#54825=CARTESIAN_POINT('',(0.0288,0.1152,0.13));
#54826=CARTESIAN_POINT('',(0.0288,0.0288,0.13));
#54827=CARTESIAN_POINT('',(0.0288,-0.0576,0.13));
#54828=CARTESIAN_POINT('',(0.0288,0.1152,0.0585));
#54829=CARTESIAN_POINT('',(0.0288,0.1152,0.0585));
#54830=CARTESIAN_POINT('',(0.0288,0.0288,0.0585));
#54831=CARTESIAN_POINT('',(0.0288,-0.1152,0.0585));
#54832=CARTESIAN_POINT('',(0.0288,0.0288,0.0585));
#54833=CARTESIAN_POINT('Origin',(-0.0288,0.1152,0.0585));
#54834=CARTESIAN_POINT('',(-0.0288,0.0288,0.13));
#54835=CARTESIAN_POINT('',(-0.0288,0.1152,0.13));
#54836=CARTESIAN_POINT('',(-0.0288,0.0576,0.13));
#54837=CARTESIAN_POINT('',(-0.0288,0.0288,0.0585));
#54838=CARTESIAN_POINT('',(-0.0288,0.0288,0.0585));
#54839=CARTESIAN_POINT('',(-0.0288,0.1152,0.0585));
#54840=CARTESIAN_POINT('',(-0.0288,0.1152,0.0585));
#54841=CARTESIAN_POINT('',(-0.0288,0.1152,0.0585));
#54842=CARTESIAN_POINT('Origin',(-0.0288,0.1152,0.0585));
#54843=CARTESIAN_POINT('',(-0.0288,-0.0288,0.13));
#54844=CARTESIAN_POINT('',(-0.0288,0.0576,0.13));
#54845=CARTESIAN_POINT('',(-0.0288,-0.0288,0.0585));
#54846=CARTESIAN_POINT('',(-0.0288,0.1152,0.0585));
#54847=CARTESIAN_POINT('',(-0.0288,-0.0288,0.0585));
#54848=CARTESIAN_POINT('Origin',(0.0288,0.1152,0.0585));
#54849=CARTESIAN_POINT('',(0.0144,0.1152,0.13));
#54850=CARTESIAN_POINT('',(0.0288,0.1152,0.0585));
#54851=CARTESIAN_POINT('Origin',(0.0288,-0.1152,0.0585));
#54852=CARTESIAN_POINT('',(0.0288,-0.0288,0.13));
#54853=CARTESIAN_POINT('',(0.0288,-0.0576,0.13));
#54854=CARTESIAN_POINT('',(0.0288,-0.0288,0.0585));
#54855=CARTESIAN_POINT('',(0.0288,-0.0288,0.0585));
#54856=CARTESIAN_POINT('',(0.0288,-0.1152,0.0585));
#54857=CARTESIAN_POINT('Origin',(0.,0.,0.13));
#54858=CARTESIAN_POINT('',(-0.1275,-1.56142466891288E-17,0.13));
#54859=CARTESIAN_POINT('Origin',(0.,0.,0.13));
#54860=CARTESIAN_POINT('',(-0.1152,-0.0288,0.13));
#54861=CARTESIAN_POINT('',(-0.0576,-0.0288,0.13));
#54862=CARTESIAN_POINT('',(-0.1152,0.0288,0.13));
#54863=CARTESIAN_POINT('',(-0.1152,0.0144,0.13));
#54864=CARTESIAN_POINT('',(0.0576,0.0288,0.13));
#54865=CARTESIAN_POINT('',(0.1152,0.0288,0.13));
#54866=CARTESIAN_POINT('',(0.0576,0.0288,0.13));
#54867=CARTESIAN_POINT('',(0.1152,-0.0288,0.13));
#54868=CARTESIAN_POINT('',(0.1152,-0.0144,0.13));
#54869=CARTESIAN_POINT('',(-0.0576,-0.0288,0.13));
#54870=CARTESIAN_POINT('Origin',(-0.1152,-0.0288,0.0585));
#54871=CARTESIAN_POINT('',(-0.1152,-0.0288,0.0585));
#54872=CARTESIAN_POINT('',(-0.1152,-0.0288,0.0585));
#54873=CARTESIAN_POINT('',(-0.1152,-0.0288,0.0585));
#54874=CARTESIAN_POINT('Origin',(0.1152,0.0288,0.0585));
#54875=CARTESIAN_POINT('',(-0.1152,0.0288,0.0585));
#54876=CARTESIAN_POINT('',(-0.1152,0.0288,0.0585));
#54877=CARTESIAN_POINT('',(0.1152,0.0288,0.0585));
#54878=CARTESIAN_POINT('Origin',(0.1152,0.0288,0.0585));
#54879=CARTESIAN_POINT('',(0.1152,0.0288,0.0585));
#54880=CARTESIAN_POINT('',(0.1152,0.0288,0.0585));
#54881=CARTESIAN_POINT('',(0.1152,0.0288,0.0585));
#54882=CARTESIAN_POINT('Origin',(-0.1152,-0.0288,0.0585));
#54883=CARTESIAN_POINT('',(0.1152,-0.0288,0.0585));
#54884=CARTESIAN_POINT('',(0.1152,-0.0288,0.0585));
#54885=CARTESIAN_POINT('',(-0.1152,-0.0288,0.0585));
#54886=CARTESIAN_POINT('Origin',(-0.1152,0.0288,0.0585));
#54887=CARTESIAN_POINT('',(-0.1152,0.0288,0.0585));
#54888=CARTESIAN_POINT('Origin',(0.1152,-0.0288,0.0585));
#54889=CARTESIAN_POINT('',(0.1152,-0.0288,0.0585));
#54890=CARTESIAN_POINT('Origin',(0.,0.,0.0585));
#54891=CARTESIAN_POINT('Origin',(0.0608,0.,-0.6));
#54892=CARTESIAN_POINT('',(-0.0608,-7.44585253881591E-18,-0.6));
#54893=CARTESIAN_POINT('Origin',(0.,0.,-0.6));
#54894=CARTESIAN_POINT('Origin',(0.,0.,-0.5904));
#54895=CARTESIAN_POINT('',(-0.0704,-8.62151346599737E-18,-0.5904));
#54896=CARTESIAN_POINT('Origin',(0.16,0.,0.));
#54897=CARTESIAN_POINT('',(-0.16,-1.95943487863577E-17,0.));
#54898=CARTESIAN_POINT('Origin',(0.,0.,0.));
#54899=CARTESIAN_POINT('Origin',(0.,0.,0.039));
#54900=CARTESIAN_POINT('',(-0.16,-1.95943487863577E-17,0.078));
#54901=CARTESIAN_POINT('Origin',(0.,0.,0.078));
#54902=CARTESIAN_POINT('',(-0.16,-1.95943487863577E-17,0.039));
#54903=CARTESIAN_POINT('Origin',(0.,0.,0.104));
#54904=CARTESIAN_POINT('',(-0.14375,-1.76042977377432E-17,0.104));
#54979=UNCERTAINTY_MEASURE_WITH_UNIT(LENGTH_MEASURE(0.001),#55003,
'DISTANCE_ACCURACY_VALUE',
'Maximum model space distance between geometric entities at asserted c
onnectivities');
#54980=UNCERTAINTY_MEASURE_WITH_UNIT(LENGTH_MEASURE(0.001),#55003,
'DISTANCE_ACCURACY_VALUE',
'Maximum model space distance between geometric entities at asserted c
onnectivities');
#55001=(
GEOMETRIC_REPRESENTATION_CONTEXT(3)
GLOBAL_UNCERTAINTY_ASSIGNED_CONTEXT((#54979))
GLOBAL_UNIT_ASSIGNED_CONTEXT((#55003,#55005,#55006))
REPRESENTATION_CONTEXT('','3D')
);
#55002=(
GEOMETRIC_REPRESENTATION_CONTEXT(3)
GLOBAL_UNCERTAINTY_ASSIGNED_CONTEXT((#54980))
GLOBAL_UNIT_ASSIGNED_CONTEXT((#55003,#55005,#55006))
REPRESENTATION_CONTEXT('','3D')
);
#55003=(
LENGTH_UNIT()
NAMED_UNIT(*)
SI_UNIT(.CENTI.,.METRE.)
);
#55005=(
NAMED_UNIT(*)
PLANE_ANGLE_UNIT()
SI_UNIT($,.RADIAN.)
);
#55006=(
NAMED_UNIT(*)
SI_UNIT($,.STERADIAN.)
SOLID_ANGLE_UNIT()
);
#55027=SHAPE_DEFINITION_REPRESENTATION(#55048,#55123);
#55048=PRODUCT_DEFINITION_SHAPE('',$,#55145);
#55123=SHAPE_REPRESENTATION('',(#27074),#55001);
#55124=PRODUCT_DEFINITION_CONTEXT('part definition',#55189,'design');
#55145=PRODUCT_DEFINITION('2026-10-18-23-37-05-724',
'19_ISO_7045_M1.6x6_A2',#55166,#55124);
#55166=PRODUCT_DEFINITION_FORMATION('',$,#55211);
#55189=APPLICATION_CONTEXT(
'Core Data for Automotive Mechanical Design Process');
#55190=PRODUCT_CONTEXT('part definition',#55189,'mechanical');
#55211=PRODUCT('2026-10-18-23-37-05-724','19_ISO_7045_M1.6x6_A2',$,(#55190));
#55394=COLOUR_RGB('Off White',0.89,0.88,0.83);
#55395=FILL_AREA_STYLE_COLOUR('',#55394);
#55396=FILL_AREA_STYLE('',(#55395));
#55397=SURFACE_STYLE_FILL_AREA(#55396);
#55398=SURFACE_SIDE_STYLE('',(#55397));
#55399=SURFACE_STYLE_USAGE(.BOTH.,#55398);
#55400=PRESENTATION_STYLE_ASSIGNMENT((#55399));
ENDSEC;
END-ISO-10303-21;
